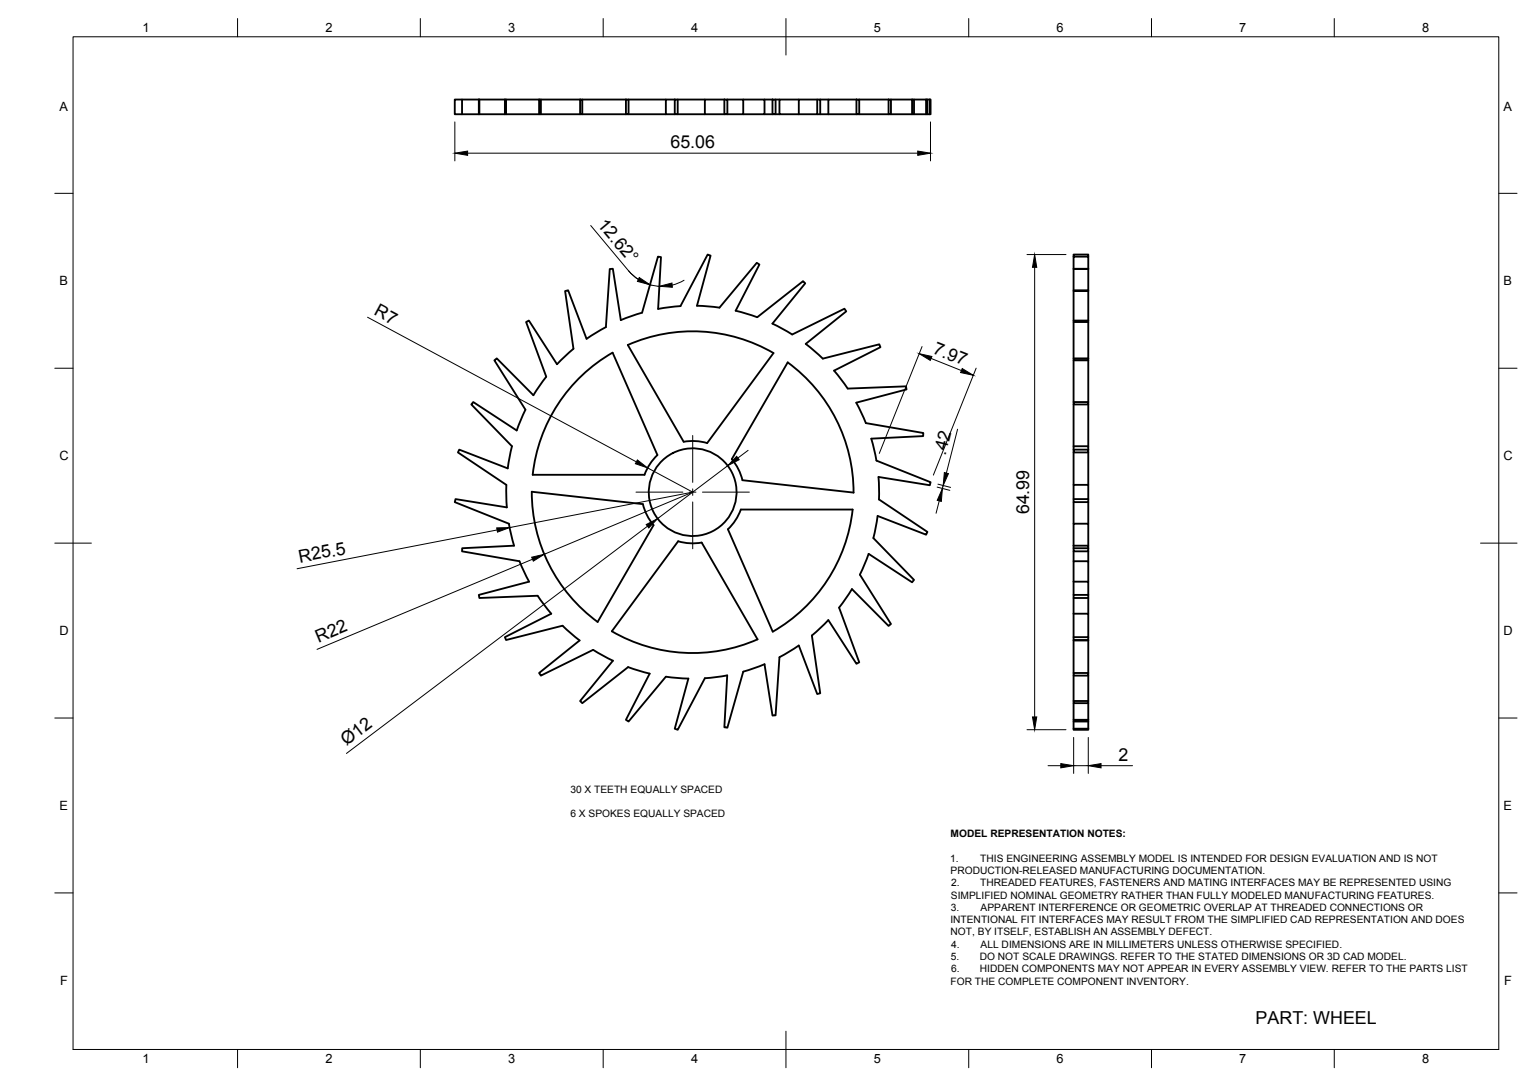
ISO-10303-21;
HEADER;
/* Generated by software containing ST-Developer
 * from STEP Tools, Inc. (www.steptools.com) 
 */

FILE_DESCRIPTION(
/* description */ (''),
/* implementation_level */ '2;1');

FILE_NAME(
/* name */ 'Wheel.step',
/* time_stamp */ '2026-10-04T15:18:51-07:00',
/* author */ (''),
/* organization */ (''),
/* preprocessor_version */ 'ST-DEVELOPER v20.2',
/* originating_system */ 'Autodesk Translation Framework v15.15.0.0',
/* authorisation */ '');

FILE_SCHEMA (('AUTOMOTIVE_DESIGN { 1 0 10303 214 3 1 1 }'));
ENDSEC;

DATA;
#10=MECHANICAL_DESIGN_GEOMETRIC_PRESENTATION_REPRESENTATION('',(#76),#9891);
#57=SHAPE_REPRESENTATION_RELATIONSHIP('SRR','None',#9928,#65);
#65=ADVANCED_BREP_SHAPE_REPRESENTATION('',(#90),#9888);
#76=STYLED_ITEM('',(#9974),#90);
#90=MANIFOLD_SOLID_BREP('Body1',#5624);
#126=FACE_BOUND('',#1015,.T.);
#127=FACE_BOUND('',#1016,.T.);
#128=FACE_BOUND('',#1017,.T.);
#129=FACE_BOUND('',#1018,.T.);
#130=FACE_BOUND('',#1019,.T.);
#131=FACE_BOUND('',#1020,.T.);
#132=FACE_BOUND('',#1021,.T.);
#133=FACE_BOUND('',#1023,.T.);
#134=FACE_BOUND('',#1024,.T.);
#135=FACE_BOUND('',#1025,.T.);
#136=FACE_BOUND('',#1026,.T.);
#137=FACE_BOUND('',#1027,.T.);
#138=FACE_BOUND('',#1028,.T.);
#139=FACE_BOUND('',#1029,.T.);
#202=PLANE('',#5949);
#203=PLANE('',#5950);
#204=PLANE('',#5951);
#205=PLANE('',#5958);
#206=PLANE('',#5959);
#207=PLANE('',#5960);
#208=PLANE('',#5964);
#209=PLANE('',#5965);
#210=PLANE('',#5966);
#211=PLANE('',#5970);
#212=PLANE('',#5971);
#213=PLANE('',#5972);
#214=PLANE('',#5976);
#215=PLANE('',#5977);
#216=PLANE('',#5978);
#217=PLANE('',#5982);
#218=PLANE('',#5983);
#219=PLANE('',#5984);
#220=PLANE('',#5991);
#221=PLANE('',#5992);
#222=PLANE('',#5993);
#223=PLANE('',#5994);
#224=PLANE('',#5995);
#225=PLANE('',#5996);
#226=PLANE('',#6000);
#227=PLANE('',#6001);
#228=PLANE('',#6002);
#229=PLANE('',#6009);
#230=PLANE('',#6010);
#231=PLANE('',#6011);
#232=PLANE('',#6018);
#233=PLANE('',#6019);
#234=PLANE('',#6020);
#235=PLANE('',#6021);
#236=PLANE('',#6022);
#237=PLANE('',#6023);
#238=PLANE('',#6024);
#239=PLANE('',#6025);
#240=PLANE('',#6026);
#241=PLANE('',#6030);
#242=PLANE('',#6031);
#243=PLANE('',#6032);
#244=PLANE('',#6036);
#245=PLANE('',#6037);
#246=PLANE('',#6038);
#247=PLANE('',#6045);
#248=PLANE('',#6046);
#249=PLANE('',#6047);
#250=PLANE('',#6051);
#251=PLANE('',#6052);
#252=PLANE('',#6053);
#253=PLANE('',#6057);
#254=PLANE('',#6058);
#255=PLANE('',#6059);
#256=PLANE('',#6060);
#257=PLANE('',#6061);
#258=PLANE('',#6062);
#259=PLANE('',#6069);
#260=PLANE('',#6070);
#261=PLANE('',#6071);
#262=PLANE('',#6072);
#263=PLANE('',#6073);
#264=PLANE('',#6074);
#265=PLANE('',#6081);
#266=PLANE('',#6082);
#267=PLANE('',#6083);
#268=PLANE('',#6084);
#269=PLANE('',#6085);
#270=PLANE('',#6086);
#271=PLANE('',#6093);
#272=PLANE('',#6094);
#273=PLANE('',#6095);
#274=PLANE('',#6099);
#275=PLANE('',#6100);
#276=PLANE('',#6101);
#277=PLANE('',#6105);
#278=PLANE('',#6106);
#279=PLANE('',#6107);
#280=PLANE('',#6111);
#281=PLANE('',#6112);
#282=PLANE('',#6113);
#283=PLANE('',#6120);
#284=PLANE('',#6121);
#285=PLANE('',#6122);
#286=PLANE('',#6123);
#287=PLANE('',#6124);
#288=PLANE('',#6125);
#289=PLANE('',#6126);
#290=PLANE('',#6127);
#291=PLANE('',#6128);
#292=PLANE('',#6129);
#293=PLANE('',#6130);
#294=PLANE('',#6143);
#295=PLANE('',#6144);
#296=PLANE('',#6151);
#297=PLANE('',#6152);
#298=PLANE('',#6159);
#299=PLANE('',#6160);
#300=PLANE('',#6167);
#301=PLANE('',#6168);
#302=PLANE('',#6175);
#303=PLANE('',#6176);
#304=PLANE('',#6180);
#305=PLANE('',#6181);
#509=FACE_OUTER_BOUND('',#869,.T.);
#510=FACE_OUTER_BOUND('',#870,.T.);
#511=FACE_OUTER_BOUND('',#871,.T.);
#512=FACE_OUTER_BOUND('',#872,.T.);
#513=FACE_OUTER_BOUND('',#873,.T.);
#514=FACE_OUTER_BOUND('',#874,.T.);
#515=FACE_OUTER_BOUND('',#875,.T.);
#516=FACE_OUTER_BOUND('',#876,.T.);
#517=FACE_OUTER_BOUND('',#877,.T.);
#518=FACE_OUTER_BOUND('',#878,.T.);
#519=FACE_OUTER_BOUND('',#879,.T.);
#520=FACE_OUTER_BOUND('',#880,.T.);
#521=FACE_OUTER_BOUND('',#881,.T.);
#522=FACE_OUTER_BOUND('',#882,.T.);
#523=FACE_OUTER_BOUND('',#883,.T.);
#524=FACE_OUTER_BOUND('',#884,.T.);
#525=FACE_OUTER_BOUND('',#885,.T.);
#526=FACE_OUTER_BOUND('',#886,.T.);
#527=FACE_OUTER_BOUND('',#887,.T.);
#528=FACE_OUTER_BOUND('',#888,.T.);
#529=FACE_OUTER_BOUND('',#889,.T.);
#530=FACE_OUTER_BOUND('',#890,.T.);
#531=FACE_OUTER_BOUND('',#891,.T.);
#532=FACE_OUTER_BOUND('',#892,.T.);
#533=FACE_OUTER_BOUND('',#893,.T.);
#534=FACE_OUTER_BOUND('',#894,.T.);
#535=FACE_OUTER_BOUND('',#895,.T.);
#536=FACE_OUTER_BOUND('',#896,.T.);
#537=FACE_OUTER_BOUND('',#897,.T.);
#538=FACE_OUTER_BOUND('',#898,.T.);
#539=FACE_OUTER_BOUND('',#899,.T.);
#540=FACE_OUTER_BOUND('',#900,.T.);
#541=FACE_OUTER_BOUND('',#901,.T.);
#542=FACE_OUTER_BOUND('',#902,.T.);
#543=FACE_OUTER_BOUND('',#903,.T.);
#544=FACE_OUTER_BOUND('',#904,.T.);
#545=FACE_OUTER_BOUND('',#905,.T.);
#546=FACE_OUTER_BOUND('',#906,.T.);
#547=FACE_OUTER_BOUND('',#907,.T.);
#548=FACE_OUTER_BOUND('',#908,.T.);
#549=FACE_OUTER_BOUND('',#909,.T.);
#550=FACE_OUTER_BOUND('',#910,.T.);
#551=FACE_OUTER_BOUND('',#911,.T.);
#552=FACE_OUTER_BOUND('',#912,.T.);
#553=FACE_OUTER_BOUND('',#913,.T.);
#554=FACE_OUTER_BOUND('',#914,.T.);
#555=FACE_OUTER_BOUND('',#915,.T.);
#556=FACE_OUTER_BOUND('',#916,.T.);
#557=FACE_OUTER_BOUND('',#917,.T.);
#558=FACE_OUTER_BOUND('',#918,.T.);
#559=FACE_OUTER_BOUND('',#919,.T.);
#560=FACE_OUTER_BOUND('',#920,.T.);
#561=FACE_OUTER_BOUND('',#921,.T.);
#562=FACE_OUTER_BOUND('',#922,.T.);
#563=FACE_OUTER_BOUND('',#923,.T.);
#564=FACE_OUTER_BOUND('',#924,.T.);
#565=FACE_OUTER_BOUND('',#925,.T.);
#566=FACE_OUTER_BOUND('',#926,.T.);
#567=FACE_OUTER_BOUND('',#927,.T.);
#568=FACE_OUTER_BOUND('',#928,.T.);
#569=FACE_OUTER_BOUND('',#929,.T.);
#570=FACE_OUTER_BOUND('',#930,.T.);
#571=FACE_OUTER_BOUND('',#931,.T.);
#572=FACE_OUTER_BOUND('',#932,.T.);
#573=FACE_OUTER_BOUND('',#933,.T.);
#574=FACE_OUTER_BOUND('',#934,.T.);
#575=FACE_OUTER_BOUND('',#935,.T.);
#576=FACE_OUTER_BOUND('',#936,.T.);
#577=FACE_OUTER_BOUND('',#937,.T.);
#578=FACE_OUTER_BOUND('',#938,.T.);
#579=FACE_OUTER_BOUND('',#939,.T.);
#580=FACE_OUTER_BOUND('',#940,.T.);
#581=FACE_OUTER_BOUND('',#941,.T.);
#582=FACE_OUTER_BOUND('',#942,.T.);
#583=FACE_OUTER_BOUND('',#943,.T.);
#584=FACE_OUTER_BOUND('',#944,.T.);
#585=FACE_OUTER_BOUND('',#945,.T.);
#586=FACE_OUTER_BOUND('',#946,.T.);
#587=FACE_OUTER_BOUND('',#947,.T.);
#588=FACE_OUTER_BOUND('',#948,.T.);
#589=FACE_OUTER_BOUND('',#949,.T.);
#590=FACE_OUTER_BOUND('',#950,.T.);
#591=FACE_OUTER_BOUND('',#951,.T.);
#592=FACE_OUTER_BOUND('',#952,.T.);
#593=FACE_OUTER_BOUND('',#953,.T.);
#594=FACE_OUTER_BOUND('',#954,.T.);
#595=FACE_OUTER_BOUND('',#955,.T.);
#596=FACE_OUTER_BOUND('',#956,.T.);
#597=FACE_OUTER_BOUND('',#957,.T.);
#598=FACE_OUTER_BOUND('',#958,.T.);
#599=FACE_OUTER_BOUND('',#959,.T.);
#600=FACE_OUTER_BOUND('',#960,.T.);
#601=FACE_OUTER_BOUND('',#961,.T.);
#602=FACE_OUTER_BOUND('',#962,.T.);
#603=FACE_OUTER_BOUND('',#963,.T.);
#604=FACE_OUTER_BOUND('',#964,.T.);
#605=FACE_OUTER_BOUND('',#965,.T.);
#606=FACE_OUTER_BOUND('',#966,.T.);
#607=FACE_OUTER_BOUND('',#967,.T.);
#608=FACE_OUTER_BOUND('',#968,.T.);
#609=FACE_OUTER_BOUND('',#969,.T.);
#610=FACE_OUTER_BOUND('',#970,.T.);
#611=FACE_OUTER_BOUND('',#971,.T.);
#612=FACE_OUTER_BOUND('',#972,.T.);
#613=FACE_OUTER_BOUND('',#973,.T.);
#614=FACE_OUTER_BOUND('',#974,.T.);
#615=FACE_OUTER_BOUND('',#975,.T.);
#616=FACE_OUTER_BOUND('',#976,.T.);
#617=FACE_OUTER_BOUND('',#977,.T.);
#618=FACE_OUTER_BOUND('',#978,.T.);
#619=FACE_OUTER_BOUND('',#979,.T.);
#620=FACE_OUTER_BOUND('',#980,.T.);
#621=FACE_OUTER_BOUND('',#981,.T.);
#622=FACE_OUTER_BOUND('',#982,.T.);
#623=FACE_OUTER_BOUND('',#983,.T.);
#624=FACE_OUTER_BOUND('',#984,.T.);
#625=FACE_OUTER_BOUND('',#985,.T.);
#626=FACE_OUTER_BOUND('',#986,.T.);
#627=FACE_OUTER_BOUND('',#987,.T.);
#628=FACE_OUTER_BOUND('',#988,.T.);
#629=FACE_OUTER_BOUND('',#989,.T.);
#630=FACE_OUTER_BOUND('',#990,.T.);
#631=FACE_OUTER_BOUND('',#991,.T.);
#632=FACE_OUTER_BOUND('',#992,.T.);
#633=FACE_OUTER_BOUND('',#993,.T.);
#634=FACE_OUTER_BOUND('',#994,.T.);
#635=FACE_OUTER_BOUND('',#995,.T.);
#636=FACE_OUTER_BOUND('',#996,.T.);
#637=FACE_OUTER_BOUND('',#997,.T.);
#638=FACE_OUTER_BOUND('',#998,.T.);
#639=FACE_OUTER_BOUND('',#999,.T.);
#640=FACE_OUTER_BOUND('',#1000,.T.);
#641=FACE_OUTER_BOUND('',#1001,.T.);
#642=FACE_OUTER_BOUND('',#1002,.T.);
#643=FACE_OUTER_BOUND('',#1003,.T.);
#644=FACE_OUTER_BOUND('',#1004,.T.);
#645=FACE_OUTER_BOUND('',#1005,.T.);
#646=FACE_OUTER_BOUND('',#1006,.T.);
#647=FACE_OUTER_BOUND('',#1007,.T.);
#648=FACE_OUTER_BOUND('',#1008,.T.);
#649=FACE_OUTER_BOUND('',#1009,.T.);
#650=FACE_OUTER_BOUND('',#1010,.T.);
#651=FACE_OUTER_BOUND('',#1011,.T.);
#652=FACE_OUTER_BOUND('',#1012,.T.);
#653=FACE_OUTER_BOUND('',#1013,.T.);
#654=FACE_OUTER_BOUND('',#1014,.T.);
#655=FACE_OUTER_BOUND('',#1022,.T.);
#869=EDGE_LOOP('',(#4016,#4017,#4018,#4019));
#870=EDGE_LOOP('',(#4020,#4021,#4022,#4023));
#871=EDGE_LOOP('',(#4024,#4025,#4026,#4027));
#872=EDGE_LOOP('',(#4028,#4029,#4030,#4031));
#873=EDGE_LOOP('',(#4032,#4033,#4034,#4035));
#874=EDGE_LOOP('',(#4036,#4037,#4038,#4039));
#875=EDGE_LOOP('',(#4040,#4041,#4042,#4043));
#876=EDGE_LOOP('',(#4044,#4045,#4046,#4047));
#877=EDGE_LOOP('',(#4048,#4049,#4050,#4051));
#878=EDGE_LOOP('',(#4052,#4053,#4054,#4055));
#879=EDGE_LOOP('',(#4056,#4057,#4058,#4059));
#880=EDGE_LOOP('',(#4060,#4061,#4062,#4063));
#881=EDGE_LOOP('',(#4064,#4065,#4066,#4067));
#882=EDGE_LOOP('',(#4068,#4069,#4070,#4071));
#883=EDGE_LOOP('',(#4072,#4073,#4074,#4075));
#884=EDGE_LOOP('',(#4076,#4077,#4078,#4079));
#885=EDGE_LOOP('',(#4080,#4081,#4082,#4083));
#886=EDGE_LOOP('',(#4084,#4085,#4086,#4087));
#887=EDGE_LOOP('',(#4088,#4089,#4090,#4091));
#888=EDGE_LOOP('',(#4092,#4093,#4094,#4095));
#889=EDGE_LOOP('',(#4096,#4097,#4098,#4099));
#890=EDGE_LOOP('',(#4100,#4101,#4102,#4103));
#891=EDGE_LOOP('',(#4104,#4105,#4106,#4107));
#892=EDGE_LOOP('',(#4108,#4109,#4110,#4111));
#893=EDGE_LOOP('',(#4112,#4113,#4114,#4115));
#894=EDGE_LOOP('',(#4116,#4117,#4118,#4119));
#895=EDGE_LOOP('',(#4120,#4121,#4122,#4123));
#896=EDGE_LOOP('',(#4124,#4125,#4126,#4127));
#897=EDGE_LOOP('',(#4128,#4129,#4130,#4131));
#898=EDGE_LOOP('',(#4132,#4133,#4134,#4135));
#899=EDGE_LOOP('',(#4136,#4137,#4138,#4139));
#900=EDGE_LOOP('',(#4140,#4141,#4142,#4143));
#901=EDGE_LOOP('',(#4144,#4145,#4146,#4147));
#902=EDGE_LOOP('',(#4148,#4149,#4150,#4151));
#903=EDGE_LOOP('',(#4152,#4153,#4154,#4155));
#904=EDGE_LOOP('',(#4156,#4157,#4158,#4159));
#905=EDGE_LOOP('',(#4160,#4161,#4162,#4163));
#906=EDGE_LOOP('',(#4164,#4165,#4166,#4167));
#907=EDGE_LOOP('',(#4168,#4169,#4170,#4171));
#908=EDGE_LOOP('',(#4172,#4173,#4174,#4175));
#909=EDGE_LOOP('',(#4176,#4177,#4178,#4179));
#910=EDGE_LOOP('',(#4180,#4181,#4182,#4183));
#911=EDGE_LOOP('',(#4184,#4185,#4186,#4187));
#912=EDGE_LOOP('',(#4188,#4189,#4190,#4191));
#913=EDGE_LOOP('',(#4192,#4193,#4194,#4195));
#914=EDGE_LOOP('',(#4196,#4197,#4198,#4199));
#915=EDGE_LOOP('',(#4200,#4201,#4202,#4203));
#916=EDGE_LOOP('',(#4204,#4205,#4206,#4207));
#917=EDGE_LOOP('',(#4208,#4209,#4210,#4211));
#918=EDGE_LOOP('',(#4212,#4213,#4214,#4215));
#919=EDGE_LOOP('',(#4216,#4217,#4218,#4219));
#920=EDGE_LOOP('',(#4220,#4221,#4222,#4223));
#921=EDGE_LOOP('',(#4224,#4225,#4226,#4227));
#922=EDGE_LOOP('',(#4228,#4229,#4230,#4231));
#923=EDGE_LOOP('',(#4232,#4233,#4234,#4235));
#924=EDGE_LOOP('',(#4236,#4237,#4238,#4239));
#925=EDGE_LOOP('',(#4240,#4241,#4242,#4243));
#926=EDGE_LOOP('',(#4244,#4245,#4246,#4247));
#927=EDGE_LOOP('',(#4248,#4249,#4250,#4251));
#928=EDGE_LOOP('',(#4252,#4253,#4254,#4255));
#929=EDGE_LOOP('',(#4256,#4257,#4258,#4259));
#930=EDGE_LOOP('',(#4260,#4261,#4262,#4263));
#931=EDGE_LOOP('',(#4264,#4265,#4266,#4267));
#932=EDGE_LOOP('',(#4268,#4269,#4270,#4271));
#933=EDGE_LOOP('',(#4272,#4273,#4274,#4275));
#934=EDGE_LOOP('',(#4276,#4277,#4278,#4279));
#935=EDGE_LOOP('',(#4280,#4281,#4282,#4283));
#936=EDGE_LOOP('',(#4284,#4285,#4286,#4287));
#937=EDGE_LOOP('',(#4288,#4289,#4290,#4291));
#938=EDGE_LOOP('',(#4292,#4293,#4294,#4295));
#939=EDGE_LOOP('',(#4296,#4297,#4298,#4299));
#940=EDGE_LOOP('',(#4300,#4301,#4302,#4303));
#941=EDGE_LOOP('',(#4304,#4305,#4306,#4307));
#942=EDGE_LOOP('',(#4308,#4309,#4310,#4311));
#943=EDGE_LOOP('',(#4312,#4313,#4314,#4315));
#944=EDGE_LOOP('',(#4316,#4317,#4318,#4319));
#945=EDGE_LOOP('',(#4320,#4321,#4322,#4323));
#946=EDGE_LOOP('',(#4324,#4325,#4326,#4327));
#947=EDGE_LOOP('',(#4328,#4329,#4330,#4331));
#948=EDGE_LOOP('',(#4332,#4333,#4334,#4335));
#949=EDGE_LOOP('',(#4336,#4337,#4338,#4339));
#950=EDGE_LOOP('',(#4340,#4341,#4342,#4343));
#951=EDGE_LOOP('',(#4344,#4345,#4346,#4347));
#952=EDGE_LOOP('',(#4348,#4349,#4350,#4351));
#953=EDGE_LOOP('',(#4352,#4353,#4354,#4355));
#954=EDGE_LOOP('',(#4356,#4357,#4358,#4359));
#955=EDGE_LOOP('',(#4360,#4361,#4362,#4363));
#956=EDGE_LOOP('',(#4364,#4365,#4366,#4367));
#957=EDGE_LOOP('',(#4368,#4369,#4370,#4371));
#958=EDGE_LOOP('',(#4372,#4373,#4374,#4375));
#959=EDGE_LOOP('',(#4376,#4377,#4378,#4379));
#960=EDGE_LOOP('',(#4380,#4381,#4382,#4383));
#961=EDGE_LOOP('',(#4384,#4385,#4386,#4387));
#962=EDGE_LOOP('',(#4388,#4389,#4390,#4391));
#963=EDGE_LOOP('',(#4392,#4393,#4394,#4395));
#964=EDGE_LOOP('',(#4396,#4397,#4398,#4399));
#965=EDGE_LOOP('',(#4400,#4401,#4402,#4403));
#966=EDGE_LOOP('',(#4404,#4405,#4406,#4407));
#967=EDGE_LOOP('',(#4408,#4409,#4410,#4411));
#968=EDGE_LOOP('',(#4412,#4413,#4414,#4415));
#969=EDGE_LOOP('',(#4416,#4417,#4418,#4419));
#970=EDGE_LOOP('',(#4420,#4421,#4422,#4423));
#971=EDGE_LOOP('',(#4424,#4425,#4426,#4427));
#972=EDGE_LOOP('',(#4428,#4429,#4430,#4431));
#973=EDGE_LOOP('',(#4432,#4433,#4434,#4435));
#974=EDGE_LOOP('',(#4436,#4437,#4438,#4439));
#975=EDGE_LOOP('',(#4440,#4441,#4442,#4443));
#976=EDGE_LOOP('',(#4444,#4445,#4446,#4447));
#977=EDGE_LOOP('',(#4448,#4449,#4450,#4451));
#978=EDGE_LOOP('',(#4452,#4453,#4454,#4455));
#979=EDGE_LOOP('',(#4456,#4457,#4458,#4459));
#980=EDGE_LOOP('',(#4460,#4461,#4462,#4463));
#981=EDGE_LOOP('',(#4464,#4465,#4466,#4467));
#982=EDGE_LOOP('',(#4468,#4469,#4470,#4471));
#983=EDGE_LOOP('',(#4472,#4473,#4474,#4475));
#984=EDGE_LOOP('',(#4476,#4477,#4478,#4479));
#985=EDGE_LOOP('',(#4480,#4481,#4482,#4483));
#986=EDGE_LOOP('',(#4484,#4485,#4486,#4487));
#987=EDGE_LOOP('',(#4488,#4489,#4490,#4491));
#988=EDGE_LOOP('',(#4492,#4493,#4494,#4495));
#989=EDGE_LOOP('',(#4496,#4497,#4498,#4499));
#990=EDGE_LOOP('',(#4500,#4501,#4502,#4503));
#991=EDGE_LOOP('',(#4504,#4505,#4506,#4507));
#992=EDGE_LOOP('',(#4508,#4509,#4510,#4511));
#993=EDGE_LOOP('',(#4512,#4513,#4514,#4515));
#994=EDGE_LOOP('',(#4516,#4517,#4518,#4519));
#995=EDGE_LOOP('',(#4520,#4521,#4522,#4523));
#996=EDGE_LOOP('',(#4524,#4525,#4526,#4527));
#997=EDGE_LOOP('',(#4528,#4529,#4530,#4531));
#998=EDGE_LOOP('',(#4532,#4533,#4534,#4535));
#999=EDGE_LOOP('',(#4536,#4537,#4538,#4539));
#1000=EDGE_LOOP('',(#4540,#4541,#4542,#4543));
#1001=EDGE_LOOP('',(#4544,#4545,#4546,#4547));
#1002=EDGE_LOOP('',(#4548,#4549,#4550,#4551));
#1003=EDGE_LOOP('',(#4552,#4553,#4554,#4555));
#1004=EDGE_LOOP('',(#4556,#4557,#4558,#4559));
#1005=EDGE_LOOP('',(#4560,#4561,#4562,#4563));
#1006=EDGE_LOOP('',(#4564,#4565,#4566,#4567));
#1007=EDGE_LOOP('',(#4568,#4569,#4570,#4571));
#1008=EDGE_LOOP('',(#4572,#4573,#4574,#4575));
#1009=EDGE_LOOP('',(#4576,#4577,#4578,#4579));
#1010=EDGE_LOOP('',(#4580,#4581,#4582,#4583));
#1011=EDGE_LOOP('',(#4584,#4585,#4586,#4587));
#1012=EDGE_LOOP('',(#4588,#4589,#4590,#4591));
#1013=EDGE_LOOP('',(#4592,#4593,#4594,#4595));
#1014=EDGE_LOOP('',(#4596,#4597,#4598,#4599,#4600,#4601,#4602,#4603,#4604,
#4605,#4606,#4607,#4608,#4609,#4610,#4611,#4612,#4613,#4614,#4615,#4616,
#4617,#4618,#4619,#4620,#4621,#4622,#4623,#4624,#4625,#4626,#4627,#4628,
#4629,#4630,#4631,#4632,#4633,#4634,#4635,#4636,#4637,#4638,#4639,#4640,
#4641,#4642,#4643,#4644,#4645,#4646,#4647,#4648,#4649,#4650,#4651,#4652,
#4653,#4654,#4655,#4656,#4657,#4658,#4659,#4660,#4661,#4662,#4663,#4664,
#4665,#4666,#4667,#4668,#4669,#4670,#4671,#4672,#4673,#4674,#4675,#4676,
#4677,#4678,#4679,#4680,#4681,#4682,#4683,#4684,#4685,#4686,#4687,#4688,
#4689,#4690,#4691,#4692,#4693,#4694,#4695,#4696,#4697,#4698,#4699,#4700,
#4701,#4702,#4703,#4704,#4705,#4706,#4707,#4708,#4709,#4710,#4711,#4712,
#4713,#4714,#4715));
#1015=EDGE_LOOP('',(#4716,#4717,#4718,#4719));
#1016=EDGE_LOOP('',(#4720,#4721,#4722,#4723));
#1017=EDGE_LOOP('',(#4724,#4725,#4726,#4727));
#1018=EDGE_LOOP('',(#4728,#4729,#4730,#4731));
#1019=EDGE_LOOP('',(#4732,#4733,#4734,#4735));
#1020=EDGE_LOOP('',(#4736));
#1021=EDGE_LOOP('',(#4737,#4738,#4739,#4740));
#1022=EDGE_LOOP('',(#4741,#4742,#4743,#4744,#4745,#4746,#4747,#4748,#4749,
#4750,#4751,#4752,#4753,#4754,#4755,#4756,#4757,#4758,#4759,#4760,#4761,
#4762,#4763,#4764,#4765,#4766,#4767,#4768,#4769,#4770,#4771,#4772,#4773,
#4774,#4775,#4776,#4777,#4778,#4779,#4780,#4781,#4782,#4783,#4784,#4785,
#4786,#4787,#4788,#4789,#4790,#4791,#4792,#4793,#4794,#4795,#4796,#4797,
#4798,#4799,#4800,#4801,#4802,#4803,#4804,#4805,#4806,#4807,#4808,#4809,
#4810,#4811,#4812,#4813,#4814,#4815,#4816,#4817,#4818,#4819,#4820,#4821,
#4822,#4823,#4824,#4825,#4826,#4827,#4828,#4829,#4830,#4831,#4832,#4833,
#4834,#4835,#4836,#4837,#4838,#4839,#4840,#4841,#4842,#4843,#4844,#4845,
#4846,#4847,#4848,#4849,#4850,#4851,#4852,#4853,#4854,#4855,#4856,#4857,
#4858,#4859,#4860));
#1023=EDGE_LOOP('',(#4861,#4862,#4863,#4864));
#1024=EDGE_LOOP('',(#4865,#4866,#4867,#4868));
#1025=EDGE_LOOP('',(#4869,#4870,#4871,#4872));
#1026=EDGE_LOOP('',(#4873,#4874,#4875,#4876));
#1027=EDGE_LOOP('',(#4877,#4878,#4879,#4880));
#1028=EDGE_LOOP('',(#4881));
#1029=EDGE_LOOP('',(#4882,#4883,#4884,#4885));
#1187=LINE('',#8656,#1651);
#1188=LINE('',#8658,#1652);
#1189=LINE('',#8660,#1653);
#1190=LINE('',#8661,#1654);
#1191=LINE('',#8664,#1655);
#1192=LINE('',#8666,#1656);
#1193=LINE('',#8667,#1657);
#1194=LINE('',#8670,#1658);
#1195=LINE('',#8672,#1659);
#1196=LINE('',#8673,#1660);
#1197=LINE('',#8678,#1661);
#1198=LINE('',#8684,#1662);
#1199=LINE('',#8689,#1663);
#1200=LINE('',#8691,#1664);
#1201=LINE('',#8693,#1665);
#1202=LINE('',#8694,#1666);
#1203=LINE('',#8697,#1667);
#1204=LINE('',#8699,#1668);
#1205=LINE('',#8700,#1669);
#1206=LINE('',#8702,#1670);
#1207=LINE('',#8703,#1671);
#1208=LINE('',#8708,#1672);
#1209=LINE('',#8713,#1673);
#1210=LINE('',#8715,#1674);
#1211=LINE('',#8717,#1675);
#1212=LINE('',#8718,#1676);
#1213=LINE('',#8721,#1677);
#1214=LINE('',#8723,#1678);
#1215=LINE('',#8724,#1679);
#1216=LINE('',#8726,#1680);
#1217=LINE('',#8727,#1681);
#1218=LINE('',#8732,#1682);
#1219=LINE('',#8737,#1683);
#1220=LINE('',#8739,#1684);
#1221=LINE('',#8741,#1685);
#1222=LINE('',#8742,#1686);
#1223=LINE('',#8745,#1687);
#1224=LINE('',#8747,#1688);
#1225=LINE('',#8748,#1689);
#1226=LINE('',#8750,#1690);
#1227=LINE('',#8751,#1691);
#1228=LINE('',#8756,#1692);
#1229=LINE('',#8761,#1693);
#1230=LINE('',#8763,#1694);
#1231=LINE('',#8765,#1695);
#1232=LINE('',#8766,#1696);
#1233=LINE('',#8769,#1697);
#1234=LINE('',#8771,#1698);
#1235=LINE('',#8772,#1699);
#1236=LINE('',#8774,#1700);
#1237=LINE('',#8775,#1701);
#1238=LINE('',#8780,#1702);
#1239=LINE('',#8785,#1703);
#1240=LINE('',#8787,#1704);
#1241=LINE('',#8789,#1705);
#1242=LINE('',#8790,#1706);
#1243=LINE('',#8793,#1707);
#1244=LINE('',#8795,#1708);
#1245=LINE('',#8796,#1709);
#1246=LINE('',#8799,#1710);
#1247=LINE('',#8801,#1711);
#1248=LINE('',#8802,#1712);
#1249=LINE('',#8807,#1713);
#1250=LINE('',#8813,#1714);
#1251=LINE('',#8818,#1715);
#1252=LINE('',#8820,#1716);
#1253=LINE('',#8822,#1717);
#1254=LINE('',#8823,#1718);
#1255=LINE('',#8825,#1719);
#1256=LINE('',#8826,#1720);
#1257=LINE('',#8828,#1721);
#1258=LINE('',#8829,#1722);
#1259=LINE('',#8833,#1723);
#1260=LINE('',#8835,#1724);
#1261=LINE('',#8837,#1725);
#1262=LINE('',#8838,#1726);
#1263=LINE('',#8841,#1727);
#1264=LINE('',#8843,#1728);
#1265=LINE('',#8844,#1729);
#1266=LINE('',#8846,#1730);
#1267=LINE('',#8847,#1731);
#1268=LINE('',#8852,#1732);
#1269=LINE('',#8857,#1733);
#1270=LINE('',#8859,#1734);
#1271=LINE('',#8861,#1735);
#1272=LINE('',#8862,#1736);
#1273=LINE('',#8865,#1737);
#1274=LINE('',#8867,#1738);
#1275=LINE('',#8868,#1739);
#1276=LINE('',#8871,#1740);
#1277=LINE('',#8873,#1741);
#1278=LINE('',#8874,#1742);
#1279=LINE('',#8879,#1743);
#1280=LINE('',#8885,#1744);
#1281=LINE('',#8890,#1745);
#1282=LINE('',#8892,#1746);
#1283=LINE('',#8894,#1747);
#1284=LINE('',#8895,#1748);
#1285=LINE('',#8898,#1749);
#1286=LINE('',#8900,#1750);
#1287=LINE('',#8901,#1751);
#1288=LINE('',#8904,#1752);
#1289=LINE('',#8906,#1753);
#1290=LINE('',#8907,#1754);
#1291=LINE('',#8912,#1755);
#1292=LINE('',#8918,#1756);
#1293=LINE('',#8923,#1757);
#1294=LINE('',#8925,#1758);
#1295=LINE('',#8927,#1759);
#1296=LINE('',#8928,#1760);
#1297=LINE('',#8930,#1761);
#1298=LINE('',#8931,#1762);
#1299=LINE('',#8933,#1763);
#1300=LINE('',#8934,#1764);
#1301=LINE('',#8938,#1765);
#1302=LINE('',#8940,#1766);
#1303=LINE('',#8942,#1767);
#1304=LINE('',#8943,#1768);
#1305=LINE('',#8945,#1769);
#1306=LINE('',#8946,#1770);
#1307=LINE('',#8948,#1771);
#1308=LINE('',#8949,#1772);
#1309=LINE('',#8953,#1773);
#1310=LINE('',#8955,#1774);
#1311=LINE('',#8957,#1775);
#1312=LINE('',#8958,#1776);
#1313=LINE('',#8961,#1777);
#1314=LINE('',#8963,#1778);
#1315=LINE('',#8964,#1779);
#1316=LINE('',#8966,#1780);
#1317=LINE('',#8967,#1781);
#1318=LINE('',#8972,#1782);
#1319=LINE('',#8977,#1783);
#1320=LINE('',#8979,#1784);
#1321=LINE('',#8981,#1785);
#1322=LINE('',#8982,#1786);
#1323=LINE('',#8985,#1787);
#1324=LINE('',#8987,#1788);
#1325=LINE('',#8988,#1789);
#1326=LINE('',#8990,#1790);
#1327=LINE('',#8991,#1791);
#1328=LINE('',#8996,#1792);
#1329=LINE('',#9001,#1793);
#1330=LINE('',#9003,#1794);
#1331=LINE('',#9005,#1795);
#1332=LINE('',#9006,#1796);
#1333=LINE('',#9009,#1797);
#1334=LINE('',#9011,#1798);
#1335=LINE('',#9012,#1799);
#1336=LINE('',#9015,#1800);
#1337=LINE('',#9017,#1801);
#1338=LINE('',#9018,#1802);
#1339=LINE('',#9023,#1803);
#1340=LINE('',#9029,#1804);
#1341=LINE('',#9034,#1805);
#1342=LINE('',#9036,#1806);
#1343=LINE('',#9038,#1807);
#1344=LINE('',#9039,#1808);
#1345=LINE('',#9042,#1809);
#1346=LINE('',#9044,#1810);
#1347=LINE('',#9045,#1811);
#1348=LINE('',#9047,#1812);
#1349=LINE('',#9048,#1813);
#1350=LINE('',#9053,#1814);
#1351=LINE('',#9058,#1815);
#1352=LINE('',#9060,#1816);
#1353=LINE('',#9062,#1817);
#1354=LINE('',#9063,#1818);
#1355=LINE('',#9066,#1819);
#1356=LINE('',#9068,#1820);
#1357=LINE('',#9069,#1821);
#1358=LINE('',#9071,#1822);
#1359=LINE('',#9072,#1823);
#1360=LINE('',#9077,#1824);
#1361=LINE('',#9082,#1825);
#1362=LINE('',#9084,#1826);
#1363=LINE('',#9086,#1827);
#1364=LINE('',#9087,#1828);
#1365=LINE('',#9089,#1829);
#1366=LINE('',#9090,#1830);
#1367=LINE('',#9092,#1831);
#1368=LINE('',#9093,#1832);
#1369=LINE('',#9097,#1833);
#1370=LINE('',#9099,#1834);
#1371=LINE('',#9101,#1835);
#1372=LINE('',#9102,#1836);
#1373=LINE('',#9105,#1837);
#1374=LINE('',#9107,#1838);
#1375=LINE('',#9108,#1839);
#1376=LINE('',#9111,#1840);
#1377=LINE('',#9113,#1841);
#1378=LINE('',#9114,#1842);
#1379=LINE('',#9119,#1843);
#1380=LINE('',#9125,#1844);
#1381=LINE('',#9130,#1845);
#1382=LINE('',#9132,#1846);
#1383=LINE('',#9134,#1847);
#1384=LINE('',#9135,#1848);
#1385=LINE('',#9137,#1849);
#1386=LINE('',#9138,#1850);
#1387=LINE('',#9140,#1851);
#1388=LINE('',#9141,#1852);
#1389=LINE('',#9145,#1853);
#1390=LINE('',#9147,#1854);
#1391=LINE('',#9149,#1855);
#1392=LINE('',#9150,#1856);
#1393=LINE('',#9153,#1857);
#1394=LINE('',#9155,#1858);
#1395=LINE('',#9156,#1859);
#1396=LINE('',#9159,#1860);
#1397=LINE('',#9161,#1861);
#1398=LINE('',#9162,#1862);
#1399=LINE('',#9167,#1863);
#1400=LINE('',#9173,#1864);
#1401=LINE('',#9178,#1865);
#1402=LINE('',#9180,#1866);
#1403=LINE('',#9182,#1867);
#1404=LINE('',#9183,#1868);
#1405=LINE('',#9185,#1869);
#1406=LINE('',#9186,#1870);
#1407=LINE('',#9188,#1871);
#1408=LINE('',#9189,#1872);
#1409=LINE('',#9193,#1873);
#1410=LINE('',#9195,#1874);
#1411=LINE('',#9197,#1875);
#1412=LINE('',#9198,#1876);
#1413=LINE('',#9201,#1877);
#1414=LINE('',#9203,#1878);
#1415=LINE('',#9204,#1879);
#1416=LINE('',#9207,#1880);
#1417=LINE('',#9209,#1881);
#1418=LINE('',#9210,#1882);
#1419=LINE('',#9215,#1883);
#1420=LINE('',#9221,#1884);
#1421=LINE('',#9226,#1885);
#1422=LINE('',#9228,#1886);
#1423=LINE('',#9230,#1887);
#1424=LINE('',#9231,#1888);
#1425=LINE('',#9234,#1889);
#1426=LINE('',#9236,#1890);
#1427=LINE('',#9237,#1891);
#1428=LINE('',#9239,#1892);
#1429=LINE('',#9240,#1893);
#1430=LINE('',#9245,#1894);
#1431=LINE('',#9250,#1895);
#1432=LINE('',#9252,#1896);
#1433=LINE('',#9254,#1897);
#1434=LINE('',#9255,#1898);
#1435=LINE('',#9258,#1899);
#1436=LINE('',#9260,#1900);
#1437=LINE('',#9261,#1901);
#1438=LINE('',#9263,#1902);
#1439=LINE('',#9264,#1903);
#1440=LINE('',#9269,#1904);
#1441=LINE('',#9274,#1905);
#1442=LINE('',#9276,#1906);
#1443=LINE('',#9278,#1907);
#1444=LINE('',#9279,#1908);
#1445=LINE('',#9281,#1909);
#1446=LINE('',#9282,#1910);
#1447=LINE('',#9285,#1911);
#1448=LINE('',#9287,#1912);
#1449=LINE('',#9288,#1913);
#1450=LINE('',#9293,#1914);
#1451=LINE('',#9298,#1915);
#1452=LINE('',#9300,#1916);
#1453=LINE('',#9302,#1917);
#1454=LINE('',#9303,#1918);
#1455=LINE('',#9306,#1919);
#1456=LINE('',#9308,#1920);
#1457=LINE('',#9309,#1921);
#1458=LINE('',#9312,#1922);
#1459=LINE('',#9314,#1923);
#1460=LINE('',#9315,#1924);
#1461=LINE('',#9320,#1925);
#1462=LINE('',#9326,#1926);
#1463=LINE('',#9331,#1927);
#1464=LINE('',#9333,#1928);
#1465=LINE('',#9335,#1929);
#1466=LINE('',#9336,#1930);
#1467=LINE('',#9338,#1931);
#1468=LINE('',#9339,#1932);
#1469=LINE('',#9341,#1933);
#1470=LINE('',#9342,#1934);
#1471=LINE('',#9346,#1935);
#1472=LINE('',#9348,#1936);
#1473=LINE('',#9350,#1937);
#1474=LINE('',#9351,#1938);
#1475=LINE('',#9353,#1939);
#1476=LINE('',#9354,#1940);
#1477=LINE('',#9356,#1941);
#1478=LINE('',#9357,#1942);
#1479=LINE('',#9361,#1943);
#1480=LINE('',#9363,#1944);
#1481=LINE('',#9365,#1945);
#1482=LINE('',#9366,#1946);
#1483=LINE('',#9368,#1947);
#1484=LINE('',#9369,#1948);
#1485=LINE('',#9371,#1949);
#1486=LINE('',#9372,#1950);
#1487=LINE('',#9376,#1951);
#1488=LINE('',#9378,#1952);
#1489=LINE('',#9380,#1953);
#1490=LINE('',#9381,#1954);
#1491=LINE('',#9385,#1955);
#1492=LINE('',#9387,#1956);
#1493=LINE('',#9389,#1957);
#1494=LINE('',#9390,#1958);
#1495=LINE('',#9395,#1959);
#1496=LINE('',#9401,#1960);
#1497=LINE('',#9407,#1961);
#1498=LINE('',#9413,#1962);
#1499=LINE('',#9416,#1963);
#1500=LINE('',#9417,#1964);
#1501=LINE('',#9421,#1965);
#1502=LINE('',#9423,#1966);
#1503=LINE('',#9425,#1967);
#1504=LINE('',#9426,#1968);
#1505=LINE('',#9431,#1969);
#1506=LINE('',#9437,#1970);
#1507=LINE('',#9440,#1971);
#1508=LINE('',#9441,#1972);
#1509=LINE('',#9445,#1973);
#1510=LINE('',#9447,#1974);
#1511=LINE('',#9449,#1975);
#1512=LINE('',#9450,#1976);
#1513=LINE('',#9455,#1977);
#1514=LINE('',#9461,#1978);
#1515=LINE('',#9464,#1979);
#1516=LINE('',#9465,#1980);
#1517=LINE('',#9469,#1981);
#1518=LINE('',#9471,#1982);
#1519=LINE('',#9473,#1983);
#1520=LINE('',#9474,#1984);
#1521=LINE('',#9479,#1985);
#1522=LINE('',#9485,#1986);
#1523=LINE('',#9488,#1987);
#1524=LINE('',#9489,#1988);
#1525=LINE('',#9493,#1989);
#1526=LINE('',#9495,#1990);
#1527=LINE('',#9497,#1991);
#1528=LINE('',#9498,#1992);
#1529=LINE('',#9503,#1993);
#1530=LINE('',#9509,#1994);
#1531=LINE('',#9512,#1995);
#1532=LINE('',#9513,#1996);
#1533=LINE('',#9515,#1997);
#1534=LINE('',#9516,#1998);
#1535=LINE('',#9521,#1999);
#1651=VECTOR('',#6888,10.);
#1652=VECTOR('',#6889,10.);
#1653=VECTOR('',#6890,10.);
#1654=VECTOR('',#6891,10.);
#1655=VECTOR('',#6894,10.);
#1656=VECTOR('',#6895,10.);
#1657=VECTOR('',#6896,10.);
#1658=VECTOR('',#6899,10.);
#1659=VECTOR('',#6900,10.);
#1660=VECTOR('',#6901,10.);
#1661=VECTOR('',#6906,10.);
#1662=VECTOR('',#6913,10.);
#1663=VECTOR('',#6918,10.);
#1664=VECTOR('',#6919,10.);
#1665=VECTOR('',#6920,10.);
#1666=VECTOR('',#6921,10.);
#1667=VECTOR('',#6924,10.);
#1668=VECTOR('',#6925,10.);
#1669=VECTOR('',#6926,10.);
#1670=VECTOR('',#6929,10.);
#1671=VECTOR('',#6930,10.);
#1672=VECTOR('',#6935,10.);
#1673=VECTOR('',#6940,10.);
#1674=VECTOR('',#6941,10.);
#1675=VECTOR('',#6942,10.);
#1676=VECTOR('',#6943,10.);
#1677=VECTOR('',#6946,10.);
#1678=VECTOR('',#6947,10.);
#1679=VECTOR('',#6948,10.);
#1680=VECTOR('',#6951,10.);
#1681=VECTOR('',#6952,10.);
#1682=VECTOR('',#6957,10.);
#1683=VECTOR('',#6962,10.);
#1684=VECTOR('',#6963,10.);
#1685=VECTOR('',#6964,10.);
#1686=VECTOR('',#6965,10.);
#1687=VECTOR('',#6968,10.);
#1688=VECTOR('',#6969,10.);
#1689=VECTOR('',#6970,10.);
#1690=VECTOR('',#6973,10.);
#1691=VECTOR('',#6974,10.);
#1692=VECTOR('',#6979,10.);
#1693=VECTOR('',#6984,10.);
#1694=VECTOR('',#6985,10.);
#1695=VECTOR('',#6986,10.);
#1696=VECTOR('',#6987,10.);
#1697=VECTOR('',#6990,10.);
#1698=VECTOR('',#6991,10.);
#1699=VECTOR('',#6992,10.);
#1700=VECTOR('',#6995,9.99999999999999);
#1701=VECTOR('',#6996,9.99999999999999);
#1702=VECTOR('',#7001,10.);
#1703=VECTOR('',#7006,10.);
#1704=VECTOR('',#7007,10.);
#1705=VECTOR('',#7008,10.);
#1706=VECTOR('',#7009,10.);
#1707=VECTOR('',#7012,10.);
#1708=VECTOR('',#7013,10.);
#1709=VECTOR('',#7014,10.);
#1710=VECTOR('',#7017,10.);
#1711=VECTOR('',#7018,10.);
#1712=VECTOR('',#7019,10.);
#1713=VECTOR('',#7024,10.);
#1714=VECTOR('',#7031,10.);
#1715=VECTOR('',#7036,9.99999999999999);
#1716=VECTOR('',#7037,10.);
#1717=VECTOR('',#7038,9.99999999999999);
#1718=VECTOR('',#7039,10.);
#1719=VECTOR('',#7042,10.);
#1720=VECTOR('',#7043,10.);
#1721=VECTOR('',#7046,10.);
#1722=VECTOR('',#7047,10.);
#1723=VECTOR('',#7050,10.);
#1724=VECTOR('',#7051,10.);
#1725=VECTOR('',#7052,10.);
#1726=VECTOR('',#7053,10.);
#1727=VECTOR('',#7056,10.);
#1728=VECTOR('',#7057,10.);
#1729=VECTOR('',#7058,10.);
#1730=VECTOR('',#7061,10.);
#1731=VECTOR('',#7062,10.);
#1732=VECTOR('',#7067,10.);
#1733=VECTOR('',#7072,10.);
#1734=VECTOR('',#7073,10.);
#1735=VECTOR('',#7074,10.);
#1736=VECTOR('',#7075,10.);
#1737=VECTOR('',#7078,9.99999999999999);
#1738=VECTOR('',#7079,9.99999999999999);
#1739=VECTOR('',#7080,10.);
#1740=VECTOR('',#7083,10.);
#1741=VECTOR('',#7084,10.);
#1742=VECTOR('',#7085,10.);
#1743=VECTOR('',#7090,10.);
#1744=VECTOR('',#7097,10.);
#1745=VECTOR('',#7102,10.);
#1746=VECTOR('',#7103,10.);
#1747=VECTOR('',#7104,10.);
#1748=VECTOR('',#7105,10.);
#1749=VECTOR('',#7108,10.);
#1750=VECTOR('',#7109,10.);
#1751=VECTOR('',#7110,10.);
#1752=VECTOR('',#7113,9.99999999999999);
#1753=VECTOR('',#7114,10.);
#1754=VECTOR('',#7115,9.99999999999999);
#1755=VECTOR('',#7120,10.);
#1756=VECTOR('',#7127,10.);
#1757=VECTOR('',#7132,10.);
#1758=VECTOR('',#7133,10.);
#1759=VECTOR('',#7134,10.);
#1760=VECTOR('',#7135,10.);
#1761=VECTOR('',#7138,10.);
#1762=VECTOR('',#7139,10.);
#1763=VECTOR('',#7142,10.);
#1764=VECTOR('',#7143,10.);
#1765=VECTOR('',#7146,10.);
#1766=VECTOR('',#7147,10.);
#1767=VECTOR('',#7148,10.);
#1768=VECTOR('',#7149,10.);
#1769=VECTOR('',#7152,10.);
#1770=VECTOR('',#7153,10.);
#1771=VECTOR('',#7156,10.);
#1772=VECTOR('',#7157,10.);
#1773=VECTOR('',#7160,10.);
#1774=VECTOR('',#7161,10.);
#1775=VECTOR('',#7162,10.);
#1776=VECTOR('',#7163,10.);
#1777=VECTOR('',#7166,10.);
#1778=VECTOR('',#7167,10.);
#1779=VECTOR('',#7168,10.);
#1780=VECTOR('',#7171,10.);
#1781=VECTOR('',#7172,10.);
#1782=VECTOR('',#7177,10.);
#1783=VECTOR('',#7182,10.);
#1784=VECTOR('',#7183,10.);
#1785=VECTOR('',#7184,10.);
#1786=VECTOR('',#7185,10.);
#1787=VECTOR('',#7188,10.);
#1788=VECTOR('',#7189,10.);
#1789=VECTOR('',#7190,10.);
#1790=VECTOR('',#7193,10.);
#1791=VECTOR('',#7194,10.);
#1792=VECTOR('',#7199,10.);
#1793=VECTOR('',#7204,10.);
#1794=VECTOR('',#7205,10.);
#1795=VECTOR('',#7206,10.);
#1796=VECTOR('',#7207,10.);
#1797=VECTOR('',#7210,10.);
#1798=VECTOR('',#7211,10.);
#1799=VECTOR('',#7212,10.);
#1800=VECTOR('',#7215,10.);
#1801=VECTOR('',#7216,10.);
#1802=VECTOR('',#7217,10.);
#1803=VECTOR('',#7222,10.);
#1804=VECTOR('',#7229,10.);
#1805=VECTOR('',#7234,10.);
#1806=VECTOR('',#7235,10.);
#1807=VECTOR('',#7236,10.);
#1808=VECTOR('',#7237,10.);
#1809=VECTOR('',#7240,10.);
#1810=VECTOR('',#7241,10.);
#1811=VECTOR('',#7242,10.);
#1812=VECTOR('',#7245,10.);
#1813=VECTOR('',#7246,10.);
#1814=VECTOR('',#7251,10.);
#1815=VECTOR('',#7256,10.);
#1816=VECTOR('',#7257,10.);
#1817=VECTOR('',#7258,10.);
#1818=VECTOR('',#7259,10.);
#1819=VECTOR('',#7262,10.);
#1820=VECTOR('',#7263,10.);
#1821=VECTOR('',#7264,10.);
#1822=VECTOR('',#7267,10.);
#1823=VECTOR('',#7268,10.);
#1824=VECTOR('',#7273,10.);
#1825=VECTOR('',#7278,10.);
#1826=VECTOR('',#7279,10.);
#1827=VECTOR('',#7280,10.);
#1828=VECTOR('',#7281,10.);
#1829=VECTOR('',#7284,10.);
#1830=VECTOR('',#7285,10.);
#1831=VECTOR('',#7288,10.);
#1832=VECTOR('',#7289,10.);
#1833=VECTOR('',#7292,10.);
#1834=VECTOR('',#7293,10.);
#1835=VECTOR('',#7294,10.);
#1836=VECTOR('',#7295,10.);
#1837=VECTOR('',#7298,10.);
#1838=VECTOR('',#7299,10.);
#1839=VECTOR('',#7300,10.);
#1840=VECTOR('',#7303,10.);
#1841=VECTOR('',#7304,10.);
#1842=VECTOR('',#7305,10.);
#1843=VECTOR('',#7310,10.);
#1844=VECTOR('',#7317,10.);
#1845=VECTOR('',#7322,10.);
#1846=VECTOR('',#7323,10.);
#1847=VECTOR('',#7324,10.);
#1848=VECTOR('',#7325,10.);
#1849=VECTOR('',#7328,10.);
#1850=VECTOR('',#7329,10.);
#1851=VECTOR('',#7332,10.);
#1852=VECTOR('',#7333,10.);
#1853=VECTOR('',#7336,10.);
#1854=VECTOR('',#7337,10.);
#1855=VECTOR('',#7338,10.);
#1856=VECTOR('',#7339,10.);
#1857=VECTOR('',#7342,10.);
#1858=VECTOR('',#7343,10.);
#1859=VECTOR('',#7344,10.);
#1860=VECTOR('',#7347,10.);
#1861=VECTOR('',#7348,10.);
#1862=VECTOR('',#7349,10.);
#1863=VECTOR('',#7354,10.);
#1864=VECTOR('',#7361,10.);
#1865=VECTOR('',#7366,10.);
#1866=VECTOR('',#7367,10.);
#1867=VECTOR('',#7368,10.);
#1868=VECTOR('',#7369,10.);
#1869=VECTOR('',#7372,10.);
#1870=VECTOR('',#7373,10.);
#1871=VECTOR('',#7376,10.);
#1872=VECTOR('',#7377,10.);
#1873=VECTOR('',#7380,10.);
#1874=VECTOR('',#7381,10.);
#1875=VECTOR('',#7382,10.);
#1876=VECTOR('',#7383,10.);
#1877=VECTOR('',#7386,10.);
#1878=VECTOR('',#7387,10.);
#1879=VECTOR('',#7388,10.);
#1880=VECTOR('',#7391,10.);
#1881=VECTOR('',#7392,10.);
#1882=VECTOR('',#7393,10.);
#1883=VECTOR('',#7398,10.);
#1884=VECTOR('',#7405,10.);
#1885=VECTOR('',#7410,10.);
#1886=VECTOR('',#7411,10.);
#1887=VECTOR('',#7412,10.);
#1888=VECTOR('',#7413,10.);
#1889=VECTOR('',#7416,10.);
#1890=VECTOR('',#7417,10.);
#1891=VECTOR('',#7418,10.);
#1892=VECTOR('',#7421,10.);
#1893=VECTOR('',#7422,10.);
#1894=VECTOR('',#7427,10.);
#1895=VECTOR('',#7432,10.);
#1896=VECTOR('',#7433,10.);
#1897=VECTOR('',#7434,10.);
#1898=VECTOR('',#7435,10.);
#1899=VECTOR('',#7438,10.);
#1900=VECTOR('',#7439,10.);
#1901=VECTOR('',#7440,10.);
#1902=VECTOR('',#7443,10.);
#1903=VECTOR('',#7444,10.);
#1904=VECTOR('',#7449,10.);
#1905=VECTOR('',#7454,10.);
#1906=VECTOR('',#7455,10.);
#1907=VECTOR('',#7456,10.);
#1908=VECTOR('',#7457,10.);
#1909=VECTOR('',#7460,10.);
#1910=VECTOR('',#7461,10.);
#1911=VECTOR('',#7464,10.);
#1912=VECTOR('',#7465,10.);
#1913=VECTOR('',#7466,10.);
#1914=VECTOR('',#7471,10.);
#1915=VECTOR('',#7476,10.);
#1916=VECTOR('',#7477,10.);
#1917=VECTOR('',#7478,10.);
#1918=VECTOR('',#7479,10.);
#1919=VECTOR('',#7482,10.);
#1920=VECTOR('',#7483,10.);
#1921=VECTOR('',#7484,10.);
#1922=VECTOR('',#7487,10.);
#1923=VECTOR('',#7488,10.);
#1924=VECTOR('',#7489,10.);
#1925=VECTOR('',#7494,10.);
#1926=VECTOR('',#7501,10.);
#1927=VECTOR('',#7506,10.);
#1928=VECTOR('',#7507,10.);
#1929=VECTOR('',#7508,10.);
#1930=VECTOR('',#7509,10.);
#1931=VECTOR('',#7512,10.);
#1932=VECTOR('',#7513,10.);
#1933=VECTOR('',#7516,10.);
#1934=VECTOR('',#7517,10.);
#1935=VECTOR('',#7520,10.);
#1936=VECTOR('',#7521,10.);
#1937=VECTOR('',#7522,10.);
#1938=VECTOR('',#7523,10.);
#1939=VECTOR('',#7526,10.);
#1940=VECTOR('',#7527,10.);
#1941=VECTOR('',#7530,10.);
#1942=VECTOR('',#7531,10.);
#1943=VECTOR('',#7534,10.);
#1944=VECTOR('',#7535,10.);
#1945=VECTOR('',#7536,10.);
#1946=VECTOR('',#7537,10.);
#1947=VECTOR('',#7540,10.);
#1948=VECTOR('',#7541,10.);
#1949=VECTOR('',#7544,10.);
#1950=VECTOR('',#7545,10.);
#1951=VECTOR('',#7548,10.);
#1952=VECTOR('',#7549,10.);
#1953=VECTOR('',#7550,10.);
#1954=VECTOR('',#7551,10.);
#1955=VECTOR('',#7554,10.);
#1956=VECTOR('',#7555,10.);
#1957=VECTOR('',#7556,10.);
#1958=VECTOR('',#7557,10.);
#1959=VECTOR('',#7562,10.);
#1960=VECTOR('',#7569,10.);
#1961=VECTOR('',#7576,10.);
#1962=VECTOR('',#7583,10.);
#1963=VECTOR('',#7588,10.);
#1964=VECTOR('',#7589,10.);
#1965=VECTOR('',#7592,10.);
#1966=VECTOR('',#7593,10.);
#1967=VECTOR('',#7594,10.);
#1968=VECTOR('',#7595,10.);
#1969=VECTOR('',#7600,10.);
#1970=VECTOR('',#7607,10.);
#1971=VECTOR('',#7612,10.);
#1972=VECTOR('',#7613,10.);
#1973=VECTOR('',#7616,10.);
#1974=VECTOR('',#7617,10.);
#1975=VECTOR('',#7618,10.);
#1976=VECTOR('',#7619,10.);
#1977=VECTOR('',#7624,10.);
#1978=VECTOR('',#7631,10.);
#1979=VECTOR('',#7636,10.);
#1980=VECTOR('',#7637,10.);
#1981=VECTOR('',#7640,10.);
#1982=VECTOR('',#7641,10.);
#1983=VECTOR('',#7642,10.);
#1984=VECTOR('',#7643,10.);
#1985=VECTOR('',#7648,10.);
#1986=VECTOR('',#7655,10.);
#1987=VECTOR('',#7660,10.);
#1988=VECTOR('',#7661,10.);
#1989=VECTOR('',#7664,10.);
#1990=VECTOR('',#7665,10.);
#1991=VECTOR('',#7666,10.);
#1992=VECTOR('',#7667,10.);
#1993=VECTOR('',#7672,10.);
#1994=VECTOR('',#7679,10.);
#1995=VECTOR('',#7684,9.99999999999999);
#1996=VECTOR('',#7685,9.99999999999999);
#1997=VECTOR('',#7688,10.);
#1998=VECTOR('',#7689,10.);
#1999=VECTOR('',#7694,6.00000000000001);
#2181=CIRCLE('',#5953,25.5);
#2182=CIRCLE('',#5954,25.5);
#2183=CIRCLE('',#5956,25.5);
#2184=CIRCLE('',#5957,25.5);
#2185=CIRCLE('',#5962,25.5);
#2186=CIRCLE('',#5963,25.5);
#2187=CIRCLE('',#5968,25.5);
#2188=CIRCLE('',#5969,25.5);
#2189=CIRCLE('',#5974,25.5);
#2190=CIRCLE('',#5975,25.5);
#2191=CIRCLE('',#5980,25.5);
#2192=CIRCLE('',#5981,25.5);
#2193=CIRCLE('',#5986,25.5);
#2194=CIRCLE('',#5987,25.5);
#2195=CIRCLE('',#5989,25.5);
#2196=CIRCLE('',#5990,25.5);
#2197=CIRCLE('',#5998,25.5);
#2198=CIRCLE('',#5999,25.5);
#2199=CIRCLE('',#6004,25.5);
#2200=CIRCLE('',#6005,25.5);
#2201=CIRCLE('',#6007,25.5);
#2202=CIRCLE('',#6008,25.5);
#2203=CIRCLE('',#6013,25.5);
#2204=CIRCLE('',#6014,25.5);
#2205=CIRCLE('',#6016,25.5);
#2206=CIRCLE('',#6017,25.5);
#2207=CIRCLE('',#6028,25.5);
#2208=CIRCLE('',#6029,25.5);
#2209=CIRCLE('',#6034,25.5);
#2210=CIRCLE('',#6035,25.5);
#2211=CIRCLE('',#6040,25.5);
#2212=CIRCLE('',#6041,25.5);
#2213=CIRCLE('',#6043,25.5);
#2214=CIRCLE('',#6044,25.5);
#2215=CIRCLE('',#6049,25.5);
#2216=CIRCLE('',#6050,25.5);
#2217=CIRCLE('',#6055,25.5);
#2218=CIRCLE('',#6056,25.5);
#2219=CIRCLE('',#6064,25.5);
#2220=CIRCLE('',#6065,25.5);
#2221=CIRCLE('',#6067,25.5);
#2222=CIRCLE('',#6068,25.5);
#2223=CIRCLE('',#6076,25.5);
#2224=CIRCLE('',#6077,25.5);
#2225=CIRCLE('',#6079,25.5);
#2226=CIRCLE('',#6080,25.5);
#2227=CIRCLE('',#6088,25.5);
#2228=CIRCLE('',#6089,25.5);
#2229=CIRCLE('',#6091,25.5);
#2230=CIRCLE('',#6092,25.5);
#2231=CIRCLE('',#6097,25.5);
#2232=CIRCLE('',#6098,25.5);
#2233=CIRCLE('',#6103,25.5);
#2234=CIRCLE('',#6104,25.5);
#2235=CIRCLE('',#6109,25.5);
#2236=CIRCLE('',#6110,25.5);
#2237=CIRCLE('',#6115,25.5);
#2238=CIRCLE('',#6116,25.5);
#2239=CIRCLE('',#6118,25.5);
#2240=CIRCLE('',#6119,25.5);
#2241=CIRCLE('',#6132,22.);
#2242=CIRCLE('',#6133,22.);
#2243=CIRCLE('',#6135,22.);
#2244=CIRCLE('',#6136,22.);
#2245=CIRCLE('',#6138,7.00000000000001);
#2246=CIRCLE('',#6139,7.00000000000001);
#2247=CIRCLE('',#6141,7.00000000000001);
#2248=CIRCLE('',#6142,7.00000000000001);
#2249=CIRCLE('',#6146,22.);
#2250=CIRCLE('',#6147,22.);
#2251=CIRCLE('',#6149,7.00000000000001);
#2252=CIRCLE('',#6150,7.00000000000001);
#2253=CIRCLE('',#6154,22.);
#2254=CIRCLE('',#6155,22.);
#2255=CIRCLE('',#6157,7.00000000000001);
#2256=CIRCLE('',#6158,7.00000000000001);
#2257=CIRCLE('',#6162,22.);
#2258=CIRCLE('',#6163,22.);
#2259=CIRCLE('',#6165,7.00000000000001);
#2260=CIRCLE('',#6166,7.00000000000001);
#2261=CIRCLE('',#6170,22.);
#2262=CIRCLE('',#6171,22.);
#2263=CIRCLE('',#6173,7.00000000000001);
#2264=CIRCLE('',#6174,7.00000000000001);
#2265=CIRCLE('',#6178,6.00000000000001);
#2266=CIRCLE('',#6179,6.00000000000001);
#2480=VERTEX_POINT('',#8654);
#2481=VERTEX_POINT('',#8655);
#2482=VERTEX_POINT('',#8657);
#2483=VERTEX_POINT('',#8659);
#2484=VERTEX_POINT('',#8663);
#2485=VERTEX_POINT('',#8665);
#2486=VERTEX_POINT('',#8669);
#2487=VERTEX_POINT('',#8671);
#2488=VERTEX_POINT('',#8675);
#2489=VERTEX_POINT('',#8677);
#2490=VERTEX_POINT('',#8681);
#2491=VERTEX_POINT('',#8683);
#2492=VERTEX_POINT('',#8687);
#2493=VERTEX_POINT('',#8688);
#2494=VERTEX_POINT('',#8690);
#2495=VERTEX_POINT('',#8692);
#2496=VERTEX_POINT('',#8696);
#2497=VERTEX_POINT('',#8698);
#2498=VERTEX_POINT('',#8705);
#2499=VERTEX_POINT('',#8707);
#2500=VERTEX_POINT('',#8711);
#2501=VERTEX_POINT('',#8712);
#2502=VERTEX_POINT('',#8714);
#2503=VERTEX_POINT('',#8716);
#2504=VERTEX_POINT('',#8720);
#2505=VERTEX_POINT('',#8722);
#2506=VERTEX_POINT('',#8729);
#2507=VERTEX_POINT('',#8731);
#2508=VERTEX_POINT('',#8735);
#2509=VERTEX_POINT('',#8736);
#2510=VERTEX_POINT('',#8738);
#2511=VERTEX_POINT('',#8740);
#2512=VERTEX_POINT('',#8744);
#2513=VERTEX_POINT('',#8746);
#2514=VERTEX_POINT('',#8753);
#2515=VERTEX_POINT('',#8755);
#2516=VERTEX_POINT('',#8759);
#2517=VERTEX_POINT('',#8760);
#2518=VERTEX_POINT('',#8762);
#2519=VERTEX_POINT('',#8764);
#2520=VERTEX_POINT('',#8768);
#2521=VERTEX_POINT('',#8770);
#2522=VERTEX_POINT('',#8777);
#2523=VERTEX_POINT('',#8779);
#2524=VERTEX_POINT('',#8783);
#2525=VERTEX_POINT('',#8784);
#2526=VERTEX_POINT('',#8786);
#2527=VERTEX_POINT('',#8788);
#2528=VERTEX_POINT('',#8792);
#2529=VERTEX_POINT('',#8794);
#2530=VERTEX_POINT('',#8798);
#2531=VERTEX_POINT('',#8800);
#2532=VERTEX_POINT('',#8804);
#2533=VERTEX_POINT('',#8806);
#2534=VERTEX_POINT('',#8810);
#2535=VERTEX_POINT('',#8812);
#2536=VERTEX_POINT('',#8816);
#2537=VERTEX_POINT('',#8817);
#2538=VERTEX_POINT('',#8819);
#2539=VERTEX_POINT('',#8821);
#2540=VERTEX_POINT('',#8831);
#2541=VERTEX_POINT('',#8832);
#2542=VERTEX_POINT('',#8834);
#2543=VERTEX_POINT('',#8836);
#2544=VERTEX_POINT('',#8840);
#2545=VERTEX_POINT('',#8842);
#2546=VERTEX_POINT('',#8849);
#2547=VERTEX_POINT('',#8851);
#2548=VERTEX_POINT('',#8855);
#2549=VERTEX_POINT('',#8856);
#2550=VERTEX_POINT('',#8858);
#2551=VERTEX_POINT('',#8860);
#2552=VERTEX_POINT('',#8864);
#2553=VERTEX_POINT('',#8866);
#2554=VERTEX_POINT('',#8870);
#2555=VERTEX_POINT('',#8872);
#2556=VERTEX_POINT('',#8876);
#2557=VERTEX_POINT('',#8878);
#2558=VERTEX_POINT('',#8882);
#2559=VERTEX_POINT('',#8884);
#2560=VERTEX_POINT('',#8888);
#2561=VERTEX_POINT('',#8889);
#2562=VERTEX_POINT('',#8891);
#2563=VERTEX_POINT('',#8893);
#2564=VERTEX_POINT('',#8897);
#2565=VERTEX_POINT('',#8899);
#2566=VERTEX_POINT('',#8903);
#2567=VERTEX_POINT('',#8905);
#2568=VERTEX_POINT('',#8909);
#2569=VERTEX_POINT('',#8911);
#2570=VERTEX_POINT('',#8915);
#2571=VERTEX_POINT('',#8917);
#2572=VERTEX_POINT('',#8921);
#2573=VERTEX_POINT('',#8922);
#2574=VERTEX_POINT('',#8924);
#2575=VERTEX_POINT('',#8926);
#2576=VERTEX_POINT('',#8936);
#2577=VERTEX_POINT('',#8937);
#2578=VERTEX_POINT('',#8939);
#2579=VERTEX_POINT('',#8941);
#2580=VERTEX_POINT('',#8951);
#2581=VERTEX_POINT('',#8952);
#2582=VERTEX_POINT('',#8954);
#2583=VERTEX_POINT('',#8956);
#2584=VERTEX_POINT('',#8960);
#2585=VERTEX_POINT('',#8962);
#2586=VERTEX_POINT('',#8969);
#2587=VERTEX_POINT('',#8971);
#2588=VERTEX_POINT('',#8975);
#2589=VERTEX_POINT('',#8976);
#2590=VERTEX_POINT('',#8978);
#2591=VERTEX_POINT('',#8980);
#2592=VERTEX_POINT('',#8984);
#2593=VERTEX_POINT('',#8986);
#2594=VERTEX_POINT('',#8993);
#2595=VERTEX_POINT('',#8995);
#2596=VERTEX_POINT('',#8999);
#2597=VERTEX_POINT('',#9000);
#2598=VERTEX_POINT('',#9002);
#2599=VERTEX_POINT('',#9004);
#2600=VERTEX_POINT('',#9008);
#2601=VERTEX_POINT('',#9010);
#2602=VERTEX_POINT('',#9014);
#2603=VERTEX_POINT('',#9016);
#2604=VERTEX_POINT('',#9020);
#2605=VERTEX_POINT('',#9022);
#2606=VERTEX_POINT('',#9026);
#2607=VERTEX_POINT('',#9028);
#2608=VERTEX_POINT('',#9032);
#2609=VERTEX_POINT('',#9033);
#2610=VERTEX_POINT('',#9035);
#2611=VERTEX_POINT('',#9037);
#2612=VERTEX_POINT('',#9041);
#2613=VERTEX_POINT('',#9043);
#2614=VERTEX_POINT('',#9050);
#2615=VERTEX_POINT('',#9052);
#2616=VERTEX_POINT('',#9056);
#2617=VERTEX_POINT('',#9057);
#2618=VERTEX_POINT('',#9059);
#2619=VERTEX_POINT('',#9061);
#2620=VERTEX_POINT('',#9065);
#2621=VERTEX_POINT('',#9067);
#2622=VERTEX_POINT('',#9074);
#2623=VERTEX_POINT('',#9076);
#2624=VERTEX_POINT('',#9080);
#2625=VERTEX_POINT('',#9081);
#2626=VERTEX_POINT('',#9083);
#2627=VERTEX_POINT('',#9085);
#2628=VERTEX_POINT('',#9095);
#2629=VERTEX_POINT('',#9096);
#2630=VERTEX_POINT('',#9098);
#2631=VERTEX_POINT('',#9100);
#2632=VERTEX_POINT('',#9104);
#2633=VERTEX_POINT('',#9106);
#2634=VERTEX_POINT('',#9110);
#2635=VERTEX_POINT('',#9112);
#2636=VERTEX_POINT('',#9116);
#2637=VERTEX_POINT('',#9118);
#2638=VERTEX_POINT('',#9122);
#2639=VERTEX_POINT('',#9124);
#2640=VERTEX_POINT('',#9128);
#2641=VERTEX_POINT('',#9129);
#2642=VERTEX_POINT('',#9131);
#2643=VERTEX_POINT('',#9133);
#2644=VERTEX_POINT('',#9143);
#2645=VERTEX_POINT('',#9144);
#2646=VERTEX_POINT('',#9146);
#2647=VERTEX_POINT('',#9148);
#2648=VERTEX_POINT('',#9152);
#2649=VERTEX_POINT('',#9154);
#2650=VERTEX_POINT('',#9158);
#2651=VERTEX_POINT('',#9160);
#2652=VERTEX_POINT('',#9164);
#2653=VERTEX_POINT('',#9166);
#2654=VERTEX_POINT('',#9170);
#2655=VERTEX_POINT('',#9172);
#2656=VERTEX_POINT('',#9176);
#2657=VERTEX_POINT('',#9177);
#2658=VERTEX_POINT('',#9179);
#2659=VERTEX_POINT('',#9181);
#2660=VERTEX_POINT('',#9191);
#2661=VERTEX_POINT('',#9192);
#2662=VERTEX_POINT('',#9194);
#2663=VERTEX_POINT('',#9196);
#2664=VERTEX_POINT('',#9200);
#2665=VERTEX_POINT('',#9202);
#2666=VERTEX_POINT('',#9206);
#2667=VERTEX_POINT('',#9208);
#2668=VERTEX_POINT('',#9212);
#2669=VERTEX_POINT('',#9214);
#2670=VERTEX_POINT('',#9218);
#2671=VERTEX_POINT('',#9220);
#2672=VERTEX_POINT('',#9224);
#2673=VERTEX_POINT('',#9225);
#2674=VERTEX_POINT('',#9227);
#2675=VERTEX_POINT('',#9229);
#2676=VERTEX_POINT('',#9233);
#2677=VERTEX_POINT('',#9235);
#2678=VERTEX_POINT('',#9242);
#2679=VERTEX_POINT('',#9244);
#2680=VERTEX_POINT('',#9248);
#2681=VERTEX_POINT('',#9249);
#2682=VERTEX_POINT('',#9251);
#2683=VERTEX_POINT('',#9253);
#2684=VERTEX_POINT('',#9257);
#2685=VERTEX_POINT('',#9259);
#2686=VERTEX_POINT('',#9266);
#2687=VERTEX_POINT('',#9268);
#2688=VERTEX_POINT('',#9272);
#2689=VERTEX_POINT('',#9273);
#2690=VERTEX_POINT('',#9275);
#2691=VERTEX_POINT('',#9277);
#2692=VERTEX_POINT('',#9284);
#2693=VERTEX_POINT('',#9286);
#2694=VERTEX_POINT('',#9290);
#2695=VERTEX_POINT('',#9292);
#2696=VERTEX_POINT('',#9296);
#2697=VERTEX_POINT('',#9297);
#2698=VERTEX_POINT('',#9299);
#2699=VERTEX_POINT('',#9301);
#2700=VERTEX_POINT('',#9305);
#2701=VERTEX_POINT('',#9307);
#2702=VERTEX_POINT('',#9311);
#2703=VERTEX_POINT('',#9313);
#2704=VERTEX_POINT('',#9317);
#2705=VERTEX_POINT('',#9319);
#2706=VERTEX_POINT('',#9323);
#2707=VERTEX_POINT('',#9325);
#2708=VERTEX_POINT('',#9329);
#2709=VERTEX_POINT('',#9330);
#2710=VERTEX_POINT('',#9332);
#2711=VERTEX_POINT('',#9334);
#2712=VERTEX_POINT('',#9344);
#2713=VERTEX_POINT('',#9345);
#2714=VERTEX_POINT('',#9347);
#2715=VERTEX_POINT('',#9349);
#2716=VERTEX_POINT('',#9359);
#2717=VERTEX_POINT('',#9360);
#2718=VERTEX_POINT('',#9362);
#2719=VERTEX_POINT('',#9364);
#2720=VERTEX_POINT('',#9374);
#2721=VERTEX_POINT('',#9375);
#2722=VERTEX_POINT('',#9377);
#2723=VERTEX_POINT('',#9379);
#2724=VERTEX_POINT('',#9383);
#2725=VERTEX_POINT('',#9384);
#2726=VERTEX_POINT('',#9386);
#2727=VERTEX_POINT('',#9388);
#2728=VERTEX_POINT('',#9392);
#2729=VERTEX_POINT('',#9394);
#2730=VERTEX_POINT('',#9398);
#2731=VERTEX_POINT('',#9400);
#2732=VERTEX_POINT('',#9404);
#2733=VERTEX_POINT('',#9406);
#2734=VERTEX_POINT('',#9410);
#2735=VERTEX_POINT('',#9412);
#2736=VERTEX_POINT('',#9419);
#2737=VERTEX_POINT('',#9420);
#2738=VERTEX_POINT('',#9422);
#2739=VERTEX_POINT('',#9424);
#2740=VERTEX_POINT('',#9428);
#2741=VERTEX_POINT('',#9430);
#2742=VERTEX_POINT('',#9434);
#2743=VERTEX_POINT('',#9436);
#2744=VERTEX_POINT('',#9443);
#2745=VERTEX_POINT('',#9444);
#2746=VERTEX_POINT('',#9446);
#2747=VERTEX_POINT('',#9448);
#2748=VERTEX_POINT('',#9452);
#2749=VERTEX_POINT('',#9454);
#2750=VERTEX_POINT('',#9458);
#2751=VERTEX_POINT('',#9460);
#2752=VERTEX_POINT('',#9467);
#2753=VERTEX_POINT('',#9468);
#2754=VERTEX_POINT('',#9470);
#2755=VERTEX_POINT('',#9472);
#2756=VERTEX_POINT('',#9476);
#2757=VERTEX_POINT('',#9478);
#2758=VERTEX_POINT('',#9482);
#2759=VERTEX_POINT('',#9484);
#2760=VERTEX_POINT('',#9491);
#2761=VERTEX_POINT('',#9492);
#2762=VERTEX_POINT('',#9494);
#2763=VERTEX_POINT('',#9496);
#2764=VERTEX_POINT('',#9500);
#2765=VERTEX_POINT('',#9502);
#2766=VERTEX_POINT('',#9506);
#2767=VERTEX_POINT('',#9508);
#2768=VERTEX_POINT('',#9518);
#2769=VERTEX_POINT('',#9520);
#3053=EDGE_CURVE('',#2480,#2481,#1187,.T.);
#3054=EDGE_CURVE('',#2480,#2482,#1188,.T.);
#3055=EDGE_CURVE('',#2483,#2482,#1189,.T.);
#3056=EDGE_CURVE('',#2481,#2483,#1190,.T.);
#3057=EDGE_CURVE('',#2481,#2484,#1191,.T.);
#3058=EDGE_CURVE('',#2485,#2483,#1192,.T.);
#3059=EDGE_CURVE('',#2484,#2485,#1193,.T.);
#3060=EDGE_CURVE('',#2480,#2486,#1194,.T.);
#3061=EDGE_CURVE('',#2487,#2486,#1195,.T.);
#3062=EDGE_CURVE('',#2482,#2487,#1196,.T.);
#3063=EDGE_CURVE('',#2488,#2485,#2181,.T.);
#3064=EDGE_CURVE('',#2488,#2489,#1197,.T.);
#3065=EDGE_CURVE('',#2489,#2484,#2182,.T.);
#3066=EDGE_CURVE('',#2486,#2490,#2183,.T.);
#3067=EDGE_CURVE('',#2490,#2491,#1198,.T.);
#3068=EDGE_CURVE('',#2487,#2491,#2184,.T.);
#3069=EDGE_CURVE('',#2492,#2493,#1199,.T.);
#3070=EDGE_CURVE('',#2492,#2494,#1200,.T.);
#3071=EDGE_CURVE('',#2495,#2494,#1201,.T.);
#3072=EDGE_CURVE('',#2493,#2495,#1202,.T.);
#3073=EDGE_CURVE('',#2493,#2496,#1203,.T.);
#3074=EDGE_CURVE('',#2497,#2495,#1204,.T.);
#3075=EDGE_CURVE('',#2496,#2497,#1205,.T.);
#3076=EDGE_CURVE('',#2492,#2489,#1206,.T.);
#3077=EDGE_CURVE('',#2494,#2488,#1207,.T.);
#3078=EDGE_CURVE('',#2498,#2497,#2185,.T.);
#3079=EDGE_CURVE('',#2498,#2499,#1208,.T.);
#3080=EDGE_CURVE('',#2499,#2496,#2186,.T.);
#3081=EDGE_CURVE('',#2500,#2501,#1209,.T.);
#3082=EDGE_CURVE('',#2500,#2502,#1210,.T.);
#3083=EDGE_CURVE('',#2503,#2502,#1211,.T.);
#3084=EDGE_CURVE('',#2501,#2503,#1212,.T.);
#3085=EDGE_CURVE('',#2501,#2504,#1213,.T.);
#3086=EDGE_CURVE('',#2505,#2503,#1214,.T.);
#3087=EDGE_CURVE('',#2504,#2505,#1215,.T.);
#3088=EDGE_CURVE('',#2500,#2499,#1216,.T.);
#3089=EDGE_CURVE('',#2502,#2498,#1217,.T.);
#3090=EDGE_CURVE('',#2506,#2505,#2187,.T.);
#3091=EDGE_CURVE('',#2506,#2507,#1218,.T.);
#3092=EDGE_CURVE('',#2507,#2504,#2188,.T.);
#3093=EDGE_CURVE('',#2508,#2509,#1219,.T.);
#3094=EDGE_CURVE('',#2508,#2510,#1220,.T.);
#3095=EDGE_CURVE('',#2511,#2510,#1221,.T.);
#3096=EDGE_CURVE('',#2509,#2511,#1222,.T.);
#3097=EDGE_CURVE('',#2509,#2512,#1223,.T.);
#3098=EDGE_CURVE('',#2513,#2511,#1224,.T.);
#3099=EDGE_CURVE('',#2512,#2513,#1225,.T.);
#3100=EDGE_CURVE('',#2508,#2507,#1226,.T.);
#3101=EDGE_CURVE('',#2510,#2506,#1227,.T.);
#3102=EDGE_CURVE('',#2514,#2513,#2189,.T.);
#3103=EDGE_CURVE('',#2514,#2515,#1228,.T.);
#3104=EDGE_CURVE('',#2515,#2512,#2190,.T.);
#3105=EDGE_CURVE('',#2516,#2517,#1229,.T.);
#3106=EDGE_CURVE('',#2516,#2518,#1230,.T.);
#3107=EDGE_CURVE('',#2519,#2518,#1231,.T.);
#3108=EDGE_CURVE('',#2517,#2519,#1232,.T.);
#3109=EDGE_CURVE('',#2517,#2520,#1233,.T.);
#3110=EDGE_CURVE('',#2521,#2519,#1234,.T.);
#3111=EDGE_CURVE('',#2520,#2521,#1235,.T.);
#3112=EDGE_CURVE('',#2516,#2515,#1236,.T.);
#3113=EDGE_CURVE('',#2518,#2514,#1237,.T.);
#3114=EDGE_CURVE('',#2522,#2521,#2191,.T.);
#3115=EDGE_CURVE('',#2522,#2523,#1238,.T.);
#3116=EDGE_CURVE('',#2523,#2520,#2192,.T.);
#3117=EDGE_CURVE('',#2524,#2525,#1239,.T.);
#3118=EDGE_CURVE('',#2524,#2526,#1240,.T.);
#3119=EDGE_CURVE('',#2527,#2526,#1241,.T.);
#3120=EDGE_CURVE('',#2525,#2527,#1242,.T.);
#3121=EDGE_CURVE('',#2525,#2528,#1243,.T.);
#3122=EDGE_CURVE('',#2529,#2527,#1244,.T.);
#3123=EDGE_CURVE('',#2528,#2529,#1245,.T.);
#3124=EDGE_CURVE('',#2524,#2530,#1246,.T.);
#3125=EDGE_CURVE('',#2531,#2530,#1247,.T.);
#3126=EDGE_CURVE('',#2526,#2531,#1248,.T.);
#3127=EDGE_CURVE('',#2532,#2529,#2193,.T.);
#3128=EDGE_CURVE('',#2532,#2533,#1249,.T.);
#3129=EDGE_CURVE('',#2533,#2528,#2194,.T.);
#3130=EDGE_CURVE('',#2530,#2534,#2195,.T.);
#3131=EDGE_CURVE('',#2534,#2535,#1250,.T.);
#3132=EDGE_CURVE('',#2531,#2535,#2196,.T.);
#3133=EDGE_CURVE('',#2536,#2537,#1251,.T.);
#3134=EDGE_CURVE('',#2536,#2538,#1252,.T.);
#3135=EDGE_CURVE('',#2539,#2538,#1253,.T.);
#3136=EDGE_CURVE('',#2537,#2539,#1254,.T.);
#3137=EDGE_CURVE('',#2537,#2534,#1255,.T.);
#3138=EDGE_CURVE('',#2535,#2539,#1256,.T.);
#3139=EDGE_CURVE('',#2536,#2523,#1257,.T.);
#3140=EDGE_CURVE('',#2538,#2522,#1258,.T.);
#3141=EDGE_CURVE('',#2540,#2541,#1259,.T.);
#3142=EDGE_CURVE('',#2540,#2542,#1260,.T.);
#3143=EDGE_CURVE('',#2543,#2542,#1261,.T.);
#3144=EDGE_CURVE('',#2541,#2543,#1262,.T.);
#3145=EDGE_CURVE('',#2541,#2544,#1263,.T.);
#3146=EDGE_CURVE('',#2545,#2543,#1264,.T.);
#3147=EDGE_CURVE('',#2544,#2545,#1265,.T.);
#3148=EDGE_CURVE('',#2540,#2533,#1266,.T.);
#3149=EDGE_CURVE('',#2542,#2532,#1267,.T.);
#3150=EDGE_CURVE('',#2546,#2545,#2197,.T.);
#3151=EDGE_CURVE('',#2546,#2547,#1268,.T.);
#3152=EDGE_CURVE('',#2547,#2544,#2198,.T.);
#3153=EDGE_CURVE('',#2548,#2549,#1269,.T.);
#3154=EDGE_CURVE('',#2548,#2550,#1270,.T.);
#3155=EDGE_CURVE('',#2551,#2550,#1271,.T.);
#3156=EDGE_CURVE('',#2549,#2551,#1272,.T.);
#3157=EDGE_CURVE('',#2549,#2552,#1273,.T.);
#3158=EDGE_CURVE('',#2553,#2551,#1274,.T.);
#3159=EDGE_CURVE('',#2552,#2553,#1275,.T.);
#3160=EDGE_CURVE('',#2548,#2554,#1276,.T.);
#3161=EDGE_CURVE('',#2555,#2554,#1277,.T.);
#3162=EDGE_CURVE('',#2550,#2555,#1278,.T.);
#3163=EDGE_CURVE('',#2556,#2553,#2199,.T.);
#3164=EDGE_CURVE('',#2556,#2557,#1279,.T.);
#3165=EDGE_CURVE('',#2557,#2552,#2200,.T.);
#3166=EDGE_CURVE('',#2554,#2558,#2201,.T.);
#3167=EDGE_CURVE('',#2558,#2559,#1280,.T.);
#3168=EDGE_CURVE('',#2555,#2559,#2202,.T.);
#3169=EDGE_CURVE('',#2560,#2561,#1281,.T.);
#3170=EDGE_CURVE('',#2560,#2562,#1282,.T.);
#3171=EDGE_CURVE('',#2563,#2562,#1283,.T.);
#3172=EDGE_CURVE('',#2561,#2563,#1284,.T.);
#3173=EDGE_CURVE('',#2561,#2564,#1285,.T.);
#3174=EDGE_CURVE('',#2565,#2563,#1286,.T.);
#3175=EDGE_CURVE('',#2564,#2565,#1287,.T.);
#3176=EDGE_CURVE('',#2560,#2566,#1288,.T.);
#3177=EDGE_CURVE('',#2567,#2566,#1289,.T.);
#3178=EDGE_CURVE('',#2562,#2567,#1290,.T.);
#3179=EDGE_CURVE('',#2568,#2565,#2203,.T.);
#3180=EDGE_CURVE('',#2568,#2569,#1291,.T.);
#3181=EDGE_CURVE('',#2569,#2564,#2204,.T.);
#3182=EDGE_CURVE('',#2566,#2570,#2205,.T.);
#3183=EDGE_CURVE('',#2570,#2571,#1292,.T.);
#3184=EDGE_CURVE('',#2567,#2571,#2206,.T.);
#3185=EDGE_CURVE('',#2572,#2573,#1293,.T.);
#3186=EDGE_CURVE('',#2572,#2574,#1294,.T.);
#3187=EDGE_CURVE('',#2575,#2574,#1295,.T.);
#3188=EDGE_CURVE('',#2573,#2575,#1296,.T.);
#3189=EDGE_CURVE('',#2573,#2570,#1297,.T.);
#3190=EDGE_CURVE('',#2571,#2575,#1298,.T.);
#3191=EDGE_CURVE('',#2572,#2557,#1299,.T.);
#3192=EDGE_CURVE('',#2574,#2556,#1300,.T.);
#3193=EDGE_CURVE('',#2576,#2577,#1301,.T.);
#3194=EDGE_CURVE('',#2576,#2578,#1302,.T.);
#3195=EDGE_CURVE('',#2579,#2578,#1303,.T.);
#3196=EDGE_CURVE('',#2577,#2579,#1304,.T.);
#3197=EDGE_CURVE('',#2577,#2558,#1305,.T.);
#3198=EDGE_CURVE('',#2559,#2579,#1306,.T.);
#3199=EDGE_CURVE('',#2576,#2547,#1307,.T.);
#3200=EDGE_CURVE('',#2578,#2546,#1308,.T.);
#3201=EDGE_CURVE('',#2580,#2581,#1309,.T.);
#3202=EDGE_CURVE('',#2580,#2582,#1310,.T.);
#3203=EDGE_CURVE('',#2583,#2582,#1311,.T.);
#3204=EDGE_CURVE('',#2581,#2583,#1312,.T.);
#3205=EDGE_CURVE('',#2581,#2584,#1313,.T.);
#3206=EDGE_CURVE('',#2585,#2583,#1314,.T.);
#3207=EDGE_CURVE('',#2584,#2585,#1315,.T.);
#3208=EDGE_CURVE('',#2580,#2569,#1316,.T.);
#3209=EDGE_CURVE('',#2582,#2568,#1317,.T.);
#3210=EDGE_CURVE('',#2586,#2585,#2207,.T.);
#3211=EDGE_CURVE('',#2586,#2587,#1318,.T.);
#3212=EDGE_CURVE('',#2587,#2584,#2208,.T.);
#3213=EDGE_CURVE('',#2588,#2589,#1319,.T.);
#3214=EDGE_CURVE('',#2588,#2590,#1320,.T.);
#3215=EDGE_CURVE('',#2591,#2590,#1321,.T.);
#3216=EDGE_CURVE('',#2589,#2591,#1322,.T.);
#3217=EDGE_CURVE('',#2589,#2592,#1323,.T.);
#3218=EDGE_CURVE('',#2593,#2591,#1324,.T.);
#3219=EDGE_CURVE('',#2592,#2593,#1325,.T.);
#3220=EDGE_CURVE('',#2588,#2587,#1326,.T.);
#3221=EDGE_CURVE('',#2590,#2586,#1327,.T.);
#3222=EDGE_CURVE('',#2594,#2593,#2209,.T.);
#3223=EDGE_CURVE('',#2594,#2595,#1328,.T.);
#3224=EDGE_CURVE('',#2595,#2592,#2210,.T.);
#3225=EDGE_CURVE('',#2596,#2597,#1329,.T.);
#3226=EDGE_CURVE('',#2596,#2598,#1330,.T.);
#3227=EDGE_CURVE('',#2599,#2598,#1331,.T.);
#3228=EDGE_CURVE('',#2597,#2599,#1332,.T.);
#3229=EDGE_CURVE('',#2597,#2600,#1333,.T.);
#3230=EDGE_CURVE('',#2601,#2599,#1334,.T.);
#3231=EDGE_CURVE('',#2600,#2601,#1335,.T.);
#3232=EDGE_CURVE('',#2596,#2602,#1336,.T.);
#3233=EDGE_CURVE('',#2603,#2602,#1337,.T.);
#3234=EDGE_CURVE('',#2598,#2603,#1338,.T.);
#3235=EDGE_CURVE('',#2604,#2601,#2211,.T.);
#3236=EDGE_CURVE('',#2604,#2605,#1339,.T.);
#3237=EDGE_CURVE('',#2605,#2600,#2212,.T.);
#3238=EDGE_CURVE('',#2602,#2606,#2213,.T.);
#3239=EDGE_CURVE('',#2606,#2607,#1340,.T.);
#3240=EDGE_CURVE('',#2603,#2607,#2214,.T.);
#3241=EDGE_CURVE('',#2608,#2609,#1341,.T.);
#3242=EDGE_CURVE('',#2608,#2610,#1342,.T.);
#3243=EDGE_CURVE('',#2611,#2610,#1343,.T.);
#3244=EDGE_CURVE('',#2609,#2611,#1344,.T.);
#3245=EDGE_CURVE('',#2609,#2612,#1345,.T.);
#3246=EDGE_CURVE('',#2613,#2611,#1346,.T.);
#3247=EDGE_CURVE('',#2612,#2613,#1347,.T.);
#3248=EDGE_CURVE('',#2608,#2595,#1348,.T.);
#3249=EDGE_CURVE('',#2610,#2594,#1349,.T.);
#3250=EDGE_CURVE('',#2614,#2613,#2215,.T.);
#3251=EDGE_CURVE('',#2614,#2615,#1350,.T.);
#3252=EDGE_CURVE('',#2615,#2612,#2216,.T.);
#3253=EDGE_CURVE('',#2616,#2617,#1351,.T.);
#3254=EDGE_CURVE('',#2616,#2618,#1352,.T.);
#3255=EDGE_CURVE('',#2619,#2618,#1353,.T.);
#3256=EDGE_CURVE('',#2617,#2619,#1354,.T.);
#3257=EDGE_CURVE('',#2617,#2620,#1355,.T.);
#3258=EDGE_CURVE('',#2621,#2619,#1356,.T.);
#3259=EDGE_CURVE('',#2620,#2621,#1357,.T.);
#3260=EDGE_CURVE('',#2616,#2615,#1358,.T.);
#3261=EDGE_CURVE('',#2618,#2614,#1359,.T.);
#3262=EDGE_CURVE('',#2622,#2621,#2217,.T.);
#3263=EDGE_CURVE('',#2622,#2623,#1360,.T.);
#3264=EDGE_CURVE('',#2623,#2620,#2218,.T.);
#3265=EDGE_CURVE('',#2624,#2625,#1361,.T.);
#3266=EDGE_CURVE('',#2624,#2626,#1362,.T.);
#3267=EDGE_CURVE('',#2627,#2626,#1363,.T.);
#3268=EDGE_CURVE('',#2625,#2627,#1364,.T.);
#3269=EDGE_CURVE('',#2625,#2606,#1365,.T.);
#3270=EDGE_CURVE('',#2607,#2627,#1366,.T.);
#3271=EDGE_CURVE('',#2624,#2623,#1367,.T.);
#3272=EDGE_CURVE('',#2626,#2622,#1368,.T.);
#3273=EDGE_CURVE('',#2628,#2629,#1369,.T.);
#3274=EDGE_CURVE('',#2628,#2630,#1370,.T.);
#3275=EDGE_CURVE('',#2631,#2630,#1371,.T.);
#3276=EDGE_CURVE('',#2629,#2631,#1372,.T.);
#3277=EDGE_CURVE('',#2629,#2632,#1373,.T.);
#3278=EDGE_CURVE('',#2633,#2631,#1374,.T.);
#3279=EDGE_CURVE('',#2632,#2633,#1375,.T.);
#3280=EDGE_CURVE('',#2628,#2634,#1376,.T.);
#3281=EDGE_CURVE('',#2635,#2634,#1377,.T.);
#3282=EDGE_CURVE('',#2630,#2635,#1378,.T.);
#3283=EDGE_CURVE('',#2636,#2633,#2219,.T.);
#3284=EDGE_CURVE('',#2636,#2637,#1379,.T.);
#3285=EDGE_CURVE('',#2637,#2632,#2220,.T.);
#3286=EDGE_CURVE('',#2634,#2638,#2221,.T.);
#3287=EDGE_CURVE('',#2638,#2639,#1380,.T.);
#3288=EDGE_CURVE('',#2635,#2639,#2222,.T.);
#3289=EDGE_CURVE('',#2640,#2641,#1381,.T.);
#3290=EDGE_CURVE('',#2640,#2642,#1382,.T.);
#3291=EDGE_CURVE('',#2643,#2642,#1383,.T.);
#3292=EDGE_CURVE('',#2641,#2643,#1384,.T.);
#3293=EDGE_CURVE('',#2641,#2638,#1385,.T.);
#3294=EDGE_CURVE('',#2639,#2643,#1386,.T.);
#3295=EDGE_CURVE('',#2640,#2605,#1387,.T.);
#3296=EDGE_CURVE('',#2642,#2604,#1388,.T.);
#3297=EDGE_CURVE('',#2644,#2645,#1389,.T.);
#3298=EDGE_CURVE('',#2644,#2646,#1390,.T.);
#3299=EDGE_CURVE('',#2647,#2646,#1391,.T.);
#3300=EDGE_CURVE('',#2645,#2647,#1392,.T.);
#3301=EDGE_CURVE('',#2645,#2648,#1393,.T.);
#3302=EDGE_CURVE('',#2649,#2647,#1394,.T.);
#3303=EDGE_CURVE('',#2648,#2649,#1395,.T.);
#3304=EDGE_CURVE('',#2644,#2650,#1396,.T.);
#3305=EDGE_CURVE('',#2651,#2650,#1397,.T.);
#3306=EDGE_CURVE('',#2646,#2651,#1398,.T.);
#3307=EDGE_CURVE('',#2652,#2649,#2223,.T.);
#3308=EDGE_CURVE('',#2652,#2653,#1399,.T.);
#3309=EDGE_CURVE('',#2653,#2648,#2224,.T.);
#3310=EDGE_CURVE('',#2650,#2654,#2225,.T.);
#3311=EDGE_CURVE('',#2654,#2655,#1400,.T.);
#3312=EDGE_CURVE('',#2651,#2655,#2226,.T.);
#3313=EDGE_CURVE('',#2656,#2657,#1401,.T.);
#3314=EDGE_CURVE('',#2656,#2658,#1402,.T.);
#3315=EDGE_CURVE('',#2659,#2658,#1403,.T.);
#3316=EDGE_CURVE('',#2657,#2659,#1404,.T.);
#3317=EDGE_CURVE('',#2657,#2490,#1405,.T.);
#3318=EDGE_CURVE('',#2491,#2659,#1406,.T.);
#3319=EDGE_CURVE('',#2656,#2653,#1407,.T.);
#3320=EDGE_CURVE('',#2658,#2652,#1408,.T.);
#3321=EDGE_CURVE('',#2660,#2661,#1409,.T.);
#3322=EDGE_CURVE('',#2660,#2662,#1410,.T.);
#3323=EDGE_CURVE('',#2663,#2662,#1411,.T.);
#3324=EDGE_CURVE('',#2661,#2663,#1412,.T.);
#3325=EDGE_CURVE('',#2661,#2664,#1413,.T.);
#3326=EDGE_CURVE('',#2665,#2663,#1414,.T.);
#3327=EDGE_CURVE('',#2664,#2665,#1415,.T.);
#3328=EDGE_CURVE('',#2660,#2666,#1416,.T.);
#3329=EDGE_CURVE('',#2667,#2666,#1417,.T.);
#3330=EDGE_CURVE('',#2662,#2667,#1418,.T.);
#3331=EDGE_CURVE('',#2668,#2665,#2227,.T.);
#3332=EDGE_CURVE('',#2668,#2669,#1419,.T.);
#3333=EDGE_CURVE('',#2669,#2664,#2228,.T.);
#3334=EDGE_CURVE('',#2666,#2670,#2229,.T.);
#3335=EDGE_CURVE('',#2670,#2671,#1420,.T.);
#3336=EDGE_CURVE('',#2667,#2671,#2230,.T.);
#3337=EDGE_CURVE('',#2672,#2673,#1421,.T.);
#3338=EDGE_CURVE('',#2672,#2674,#1422,.T.);
#3339=EDGE_CURVE('',#2675,#2674,#1423,.T.);
#3340=EDGE_CURVE('',#2673,#2675,#1424,.T.);
#3341=EDGE_CURVE('',#2673,#2676,#1425,.T.);
#3342=EDGE_CURVE('',#2677,#2675,#1426,.T.);
#3343=EDGE_CURVE('',#2676,#2677,#1427,.T.);
#3344=EDGE_CURVE('',#2672,#2669,#1428,.T.);
#3345=EDGE_CURVE('',#2674,#2668,#1429,.T.);
#3346=EDGE_CURVE('',#2678,#2677,#2231,.T.);
#3347=EDGE_CURVE('',#2678,#2679,#1430,.T.);
#3348=EDGE_CURVE('',#2679,#2676,#2232,.T.);
#3349=EDGE_CURVE('',#2680,#2681,#1431,.T.);
#3350=EDGE_CURVE('',#2680,#2682,#1432,.T.);
#3351=EDGE_CURVE('',#2683,#2682,#1433,.T.);
#3352=EDGE_CURVE('',#2681,#2683,#1434,.T.);
#3353=EDGE_CURVE('',#2681,#2684,#1435,.T.);
#3354=EDGE_CURVE('',#2685,#2683,#1436,.T.);
#3355=EDGE_CURVE('',#2684,#2685,#1437,.T.);
#3356=EDGE_CURVE('',#2680,#2679,#1438,.T.);
#3357=EDGE_CURVE('',#2682,#2678,#1439,.T.);
#3358=EDGE_CURVE('',#2686,#2685,#2233,.T.);
#3359=EDGE_CURVE('',#2686,#2687,#1440,.T.);
#3360=EDGE_CURVE('',#2687,#2684,#2234,.T.);
#3361=EDGE_CURVE('',#2688,#2689,#1441,.T.);
#3362=EDGE_CURVE('',#2688,#2690,#1442,.T.);
#3363=EDGE_CURVE('',#2691,#2690,#1443,.T.);
#3364=EDGE_CURVE('',#2689,#2691,#1444,.T.);
#3365=EDGE_CURVE('',#2689,#2670,#1445,.T.);
#3366=EDGE_CURVE('',#2671,#2691,#1446,.T.);
#3367=EDGE_CURVE('',#2688,#2692,#1447,.T.);
#3368=EDGE_CURVE('',#2693,#2692,#1448,.T.);
#3369=EDGE_CURVE('',#2690,#2693,#1449,.T.);
#3370=EDGE_CURVE('',#2692,#2694,#2235,.T.);
#3371=EDGE_CURVE('',#2694,#2695,#1450,.T.);
#3372=EDGE_CURVE('',#2693,#2695,#2236,.T.);
#3373=EDGE_CURVE('',#2696,#2697,#1451,.T.);
#3374=EDGE_CURVE('',#2696,#2698,#1452,.T.);
#3375=EDGE_CURVE('',#2699,#2698,#1453,.T.);
#3376=EDGE_CURVE('',#2697,#2699,#1454,.T.);
#3377=EDGE_CURVE('',#2697,#2700,#1455,.T.);
#3378=EDGE_CURVE('',#2701,#2699,#1456,.T.);
#3379=EDGE_CURVE('',#2700,#2701,#1457,.T.);
#3380=EDGE_CURVE('',#2696,#2702,#1458,.T.);
#3381=EDGE_CURVE('',#2703,#2702,#1459,.T.);
#3382=EDGE_CURVE('',#2698,#2703,#1460,.T.);
#3383=EDGE_CURVE('',#2704,#2701,#2237,.T.);
#3384=EDGE_CURVE('',#2704,#2705,#1461,.T.);
#3385=EDGE_CURVE('',#2705,#2700,#2238,.T.);
#3386=EDGE_CURVE('',#2702,#2706,#2239,.T.);
#3387=EDGE_CURVE('',#2706,#2707,#1462,.T.);
#3388=EDGE_CURVE('',#2703,#2707,#2240,.T.);
#3389=EDGE_CURVE('',#2708,#2709,#1463,.T.);
#3390=EDGE_CURVE('',#2708,#2710,#1464,.T.);
#3391=EDGE_CURVE('',#2711,#2710,#1465,.T.);
#3392=EDGE_CURVE('',#2709,#2711,#1466,.T.);
#3393=EDGE_CURVE('',#2709,#2694,#1467,.T.);
#3394=EDGE_CURVE('',#2695,#2711,#1468,.T.);
#3395=EDGE_CURVE('',#2708,#2705,#1469,.T.);
#3396=EDGE_CURVE('',#2710,#2704,#1470,.T.);
#3397=EDGE_CURVE('',#2712,#2713,#1471,.T.);
#3398=EDGE_CURVE('',#2712,#2714,#1472,.T.);
#3399=EDGE_CURVE('',#2715,#2714,#1473,.T.);
#3400=EDGE_CURVE('',#2713,#2715,#1474,.T.);
#3401=EDGE_CURVE('',#2713,#2706,#1475,.T.);
#3402=EDGE_CURVE('',#2707,#2715,#1476,.T.);
#3403=EDGE_CURVE('',#2712,#2637,#1477,.T.);
#3404=EDGE_CURVE('',#2714,#2636,#1478,.T.);
#3405=EDGE_CURVE('',#2716,#2717,#1479,.T.);
#3406=EDGE_CURVE('',#2716,#2718,#1480,.T.);
#3407=EDGE_CURVE('',#2719,#2718,#1481,.T.);
#3408=EDGE_CURVE('',#2717,#2719,#1482,.T.);
#3409=EDGE_CURVE('',#2717,#2654,#1483,.T.);
#3410=EDGE_CURVE('',#2655,#2719,#1484,.T.);
#3411=EDGE_CURVE('',#2716,#2687,#1485,.T.);
#3412=EDGE_CURVE('',#2718,#2686,#1486,.T.);
#3413=EDGE_CURVE('',#2720,#2721,#1487,.T.);
#3414=EDGE_CURVE('',#2722,#2720,#1488,.T.);
#3415=EDGE_CURVE('',#2723,#2722,#1489,.T.);
#3416=EDGE_CURVE('',#2721,#2723,#1490,.T.);
#3417=EDGE_CURVE('',#2724,#2725,#1491,.T.);
#3418=EDGE_CURVE('',#2726,#2725,#1492,.T.);
#3419=EDGE_CURVE('',#2727,#2726,#1493,.T.);
#3420=EDGE_CURVE('',#2724,#2727,#1494,.T.);
#3421=EDGE_CURVE('',#2728,#2723,#2241,.T.);
#3422=EDGE_CURVE('',#2728,#2729,#1495,.T.);
#3423=EDGE_CURVE('',#2729,#2721,#2242,.T.);
#3424=EDGE_CURVE('',#2725,#2730,#2243,.T.);
#3425=EDGE_CURVE('',#2730,#2731,#1496,.T.);
#3426=EDGE_CURVE('',#2726,#2731,#2244,.T.);
#3427=EDGE_CURVE('',#2732,#2727,#2245,.T.);
#3428=EDGE_CURVE('',#2732,#2733,#1497,.T.);
#3429=EDGE_CURVE('',#2733,#2724,#2246,.T.);
#3430=EDGE_CURVE('',#2720,#2734,#2247,.T.);
#3431=EDGE_CURVE('',#2734,#2735,#1498,.T.);
#3432=EDGE_CURVE('',#2722,#2735,#2248,.T.);
#3433=EDGE_CURVE('',#2733,#2730,#1499,.T.);
#3434=EDGE_CURVE('',#2731,#2732,#1500,.T.);
#3435=EDGE_CURVE('',#2736,#2737,#1501,.T.);
#3436=EDGE_CURVE('',#2738,#2737,#1502,.T.);
#3437=EDGE_CURVE('',#2739,#2738,#1503,.T.);
#3438=EDGE_CURVE('',#2736,#2739,#1504,.T.);
#3439=EDGE_CURVE('',#2737,#2740,#2249,.T.);
#3440=EDGE_CURVE('',#2740,#2741,#1505,.T.);
#3441=EDGE_CURVE('',#2738,#2741,#2250,.T.);
#3442=EDGE_CURVE('',#2742,#2739,#2251,.T.);
#3443=EDGE_CURVE('',#2742,#2743,#1506,.T.);
#3444=EDGE_CURVE('',#2743,#2736,#2252,.T.);
#3445=EDGE_CURVE('',#2743,#2740,#1507,.T.);
#3446=EDGE_CURVE('',#2741,#2742,#1508,.T.);
#3447=EDGE_CURVE('',#2744,#2745,#1509,.T.);
#3448=EDGE_CURVE('',#2746,#2745,#1510,.T.);
#3449=EDGE_CURVE('',#2747,#2746,#1511,.T.);
#3450=EDGE_CURVE('',#2744,#2747,#1512,.T.);
#3451=EDGE_CURVE('',#2745,#2748,#2253,.T.);
#3452=EDGE_CURVE('',#2748,#2749,#1513,.T.);
#3453=EDGE_CURVE('',#2746,#2749,#2254,.T.);
#3454=EDGE_CURVE('',#2750,#2747,#2255,.T.);
#3455=EDGE_CURVE('',#2750,#2751,#1514,.T.);
#3456=EDGE_CURVE('',#2751,#2744,#2256,.T.);
#3457=EDGE_CURVE('',#2751,#2748,#1515,.T.);
#3458=EDGE_CURVE('',#2749,#2750,#1516,.T.);
#3459=EDGE_CURVE('',#2752,#2753,#1517,.T.);
#3460=EDGE_CURVE('',#2754,#2753,#1518,.T.);
#3461=EDGE_CURVE('',#2755,#2754,#1519,.T.);
#3462=EDGE_CURVE('',#2752,#2755,#1520,.T.);
#3463=EDGE_CURVE('',#2753,#2756,#2257,.T.);
#3464=EDGE_CURVE('',#2756,#2757,#1521,.T.);
#3465=EDGE_CURVE('',#2754,#2757,#2258,.T.);
#3466=EDGE_CURVE('',#2758,#2755,#2259,.T.);
#3467=EDGE_CURVE('',#2758,#2759,#1522,.T.);
#3468=EDGE_CURVE('',#2759,#2752,#2260,.T.);
#3469=EDGE_CURVE('',#2759,#2756,#1523,.T.);
#3470=EDGE_CURVE('',#2757,#2758,#1524,.T.);
#3471=EDGE_CURVE('',#2760,#2761,#1525,.T.);
#3472=EDGE_CURVE('',#2762,#2761,#1526,.T.);
#3473=EDGE_CURVE('',#2763,#2762,#1527,.T.);
#3474=EDGE_CURVE('',#2760,#2763,#1528,.T.);
#3475=EDGE_CURVE('',#2761,#2764,#2261,.T.);
#3476=EDGE_CURVE('',#2764,#2765,#1529,.T.);
#3477=EDGE_CURVE('',#2762,#2765,#2262,.T.);
#3478=EDGE_CURVE('',#2766,#2763,#2263,.T.);
#3479=EDGE_CURVE('',#2766,#2767,#1530,.T.);
#3480=EDGE_CURVE('',#2767,#2760,#2264,.T.);
#3481=EDGE_CURVE('',#2767,#2764,#1531,.T.);
#3482=EDGE_CURVE('',#2765,#2766,#1532,.T.);
#3483=EDGE_CURVE('',#2734,#2729,#1533,.T.);
#3484=EDGE_CURVE('',#2735,#2728,#1534,.T.);
#3485=EDGE_CURVE('',#2768,#2768,#2265,.T.);
#3486=EDGE_CURVE('',#2768,#2769,#1535,.T.);
#3487=EDGE_CURVE('',#2769,#2769,#2266,.T.);
#4016=ORIENTED_EDGE('',*,*,#3053,.F.);
#4017=ORIENTED_EDGE('',*,*,#3054,.T.);
#4018=ORIENTED_EDGE('',*,*,#3055,.F.);
#4019=ORIENTED_EDGE('',*,*,#3056,.F.);
#4020=ORIENTED_EDGE('',*,*,#3057,.F.);
#4021=ORIENTED_EDGE('',*,*,#3056,.T.);
#4022=ORIENTED_EDGE('',*,*,#3058,.F.);
#4023=ORIENTED_EDGE('',*,*,#3059,.F.);
#4024=ORIENTED_EDGE('',*,*,#3060,.T.);
#4025=ORIENTED_EDGE('',*,*,#3061,.F.);
#4026=ORIENTED_EDGE('',*,*,#3062,.F.);
#4027=ORIENTED_EDGE('',*,*,#3054,.F.);
#4028=ORIENTED_EDGE('',*,*,#3059,.T.);
#4029=ORIENTED_EDGE('',*,*,#3063,.F.);
#4030=ORIENTED_EDGE('',*,*,#3064,.T.);
#4031=ORIENTED_EDGE('',*,*,#3065,.T.);
#4032=ORIENTED_EDGE('',*,*,#3061,.T.);
#4033=ORIENTED_EDGE('',*,*,#3066,.T.);
#4034=ORIENTED_EDGE('',*,*,#3067,.T.);
#4035=ORIENTED_EDGE('',*,*,#3068,.F.);
#4036=ORIENTED_EDGE('',*,*,#3069,.F.);
#4037=ORIENTED_EDGE('',*,*,#3070,.T.);
#4038=ORIENTED_EDGE('',*,*,#3071,.F.);
#4039=ORIENTED_EDGE('',*,*,#3072,.F.);
#4040=ORIENTED_EDGE('',*,*,#3073,.F.);
#4041=ORIENTED_EDGE('',*,*,#3072,.T.);
#4042=ORIENTED_EDGE('',*,*,#3074,.F.);
#4043=ORIENTED_EDGE('',*,*,#3075,.F.);
#4044=ORIENTED_EDGE('',*,*,#3076,.T.);
#4045=ORIENTED_EDGE('',*,*,#3064,.F.);
#4046=ORIENTED_EDGE('',*,*,#3077,.F.);
#4047=ORIENTED_EDGE('',*,*,#3070,.F.);
#4048=ORIENTED_EDGE('',*,*,#3075,.T.);
#4049=ORIENTED_EDGE('',*,*,#3078,.F.);
#4050=ORIENTED_EDGE('',*,*,#3079,.T.);
#4051=ORIENTED_EDGE('',*,*,#3080,.T.);
#4052=ORIENTED_EDGE('',*,*,#3081,.F.);
#4053=ORIENTED_EDGE('',*,*,#3082,.T.);
#4054=ORIENTED_EDGE('',*,*,#3083,.F.);
#4055=ORIENTED_EDGE('',*,*,#3084,.F.);
#4056=ORIENTED_EDGE('',*,*,#3085,.F.);
#4057=ORIENTED_EDGE('',*,*,#3084,.T.);
#4058=ORIENTED_EDGE('',*,*,#3086,.F.);
#4059=ORIENTED_EDGE('',*,*,#3087,.F.);
#4060=ORIENTED_EDGE('',*,*,#3088,.T.);
#4061=ORIENTED_EDGE('',*,*,#3079,.F.);
#4062=ORIENTED_EDGE('',*,*,#3089,.F.);
#4063=ORIENTED_EDGE('',*,*,#3082,.F.);
#4064=ORIENTED_EDGE('',*,*,#3087,.T.);
#4065=ORIENTED_EDGE('',*,*,#3090,.F.);
#4066=ORIENTED_EDGE('',*,*,#3091,.T.);
#4067=ORIENTED_EDGE('',*,*,#3092,.T.);
#4068=ORIENTED_EDGE('',*,*,#3093,.F.);
#4069=ORIENTED_EDGE('',*,*,#3094,.T.);
#4070=ORIENTED_EDGE('',*,*,#3095,.F.);
#4071=ORIENTED_EDGE('',*,*,#3096,.F.);
#4072=ORIENTED_EDGE('',*,*,#3097,.F.);
#4073=ORIENTED_EDGE('',*,*,#3096,.T.);
#4074=ORIENTED_EDGE('',*,*,#3098,.F.);
#4075=ORIENTED_EDGE('',*,*,#3099,.F.);
#4076=ORIENTED_EDGE('',*,*,#3100,.T.);
#4077=ORIENTED_EDGE('',*,*,#3091,.F.);
#4078=ORIENTED_EDGE('',*,*,#3101,.F.);
#4079=ORIENTED_EDGE('',*,*,#3094,.F.);
#4080=ORIENTED_EDGE('',*,*,#3099,.T.);
#4081=ORIENTED_EDGE('',*,*,#3102,.F.);
#4082=ORIENTED_EDGE('',*,*,#3103,.T.);
#4083=ORIENTED_EDGE('',*,*,#3104,.T.);
#4084=ORIENTED_EDGE('',*,*,#3105,.F.);
#4085=ORIENTED_EDGE('',*,*,#3106,.T.);
#4086=ORIENTED_EDGE('',*,*,#3107,.F.);
#4087=ORIENTED_EDGE('',*,*,#3108,.F.);
#4088=ORIENTED_EDGE('',*,*,#3109,.F.);
#4089=ORIENTED_EDGE('',*,*,#3108,.T.);
#4090=ORIENTED_EDGE('',*,*,#3110,.F.);
#4091=ORIENTED_EDGE('',*,*,#3111,.F.);
#4092=ORIENTED_EDGE('',*,*,#3112,.T.);
#4093=ORIENTED_EDGE('',*,*,#3103,.F.);
#4094=ORIENTED_EDGE('',*,*,#3113,.F.);
#4095=ORIENTED_EDGE('',*,*,#3106,.F.);
#4096=ORIENTED_EDGE('',*,*,#3111,.T.);
#4097=ORIENTED_EDGE('',*,*,#3114,.F.);
#4098=ORIENTED_EDGE('',*,*,#3115,.T.);
#4099=ORIENTED_EDGE('',*,*,#3116,.T.);
#4100=ORIENTED_EDGE('',*,*,#3117,.F.);
#4101=ORIENTED_EDGE('',*,*,#3118,.T.);
#4102=ORIENTED_EDGE('',*,*,#3119,.F.);
#4103=ORIENTED_EDGE('',*,*,#3120,.F.);
#4104=ORIENTED_EDGE('',*,*,#3121,.F.);
#4105=ORIENTED_EDGE('',*,*,#3120,.T.);
#4106=ORIENTED_EDGE('',*,*,#3122,.F.);
#4107=ORIENTED_EDGE('',*,*,#3123,.F.);
#4108=ORIENTED_EDGE('',*,*,#3124,.T.);
#4109=ORIENTED_EDGE('',*,*,#3125,.F.);
#4110=ORIENTED_EDGE('',*,*,#3126,.F.);
#4111=ORIENTED_EDGE('',*,*,#3118,.F.);
#4112=ORIENTED_EDGE('',*,*,#3123,.T.);
#4113=ORIENTED_EDGE('',*,*,#3127,.F.);
#4114=ORIENTED_EDGE('',*,*,#3128,.T.);
#4115=ORIENTED_EDGE('',*,*,#3129,.T.);
#4116=ORIENTED_EDGE('',*,*,#3125,.T.);
#4117=ORIENTED_EDGE('',*,*,#3130,.T.);
#4118=ORIENTED_EDGE('',*,*,#3131,.T.);
#4119=ORIENTED_EDGE('',*,*,#3132,.F.);
#4120=ORIENTED_EDGE('',*,*,#3133,.F.);
#4121=ORIENTED_EDGE('',*,*,#3134,.T.);
#4122=ORIENTED_EDGE('',*,*,#3135,.F.);
#4123=ORIENTED_EDGE('',*,*,#3136,.F.);
#4124=ORIENTED_EDGE('',*,*,#3137,.F.);
#4125=ORIENTED_EDGE('',*,*,#3136,.T.);
#4126=ORIENTED_EDGE('',*,*,#3138,.F.);
#4127=ORIENTED_EDGE('',*,*,#3131,.F.);
#4128=ORIENTED_EDGE('',*,*,#3139,.T.);
#4129=ORIENTED_EDGE('',*,*,#3115,.F.);
#4130=ORIENTED_EDGE('',*,*,#3140,.F.);
#4131=ORIENTED_EDGE('',*,*,#3134,.F.);
#4132=ORIENTED_EDGE('',*,*,#3141,.F.);
#4133=ORIENTED_EDGE('',*,*,#3142,.T.);
#4134=ORIENTED_EDGE('',*,*,#3143,.F.);
#4135=ORIENTED_EDGE('',*,*,#3144,.F.);
#4136=ORIENTED_EDGE('',*,*,#3145,.F.);
#4137=ORIENTED_EDGE('',*,*,#3144,.T.);
#4138=ORIENTED_EDGE('',*,*,#3146,.F.);
#4139=ORIENTED_EDGE('',*,*,#3147,.F.);
#4140=ORIENTED_EDGE('',*,*,#3148,.T.);
#4141=ORIENTED_EDGE('',*,*,#3128,.F.);
#4142=ORIENTED_EDGE('',*,*,#3149,.F.);
#4143=ORIENTED_EDGE('',*,*,#3142,.F.);
#4144=ORIENTED_EDGE('',*,*,#3147,.T.);
#4145=ORIENTED_EDGE('',*,*,#3150,.F.);
#4146=ORIENTED_EDGE('',*,*,#3151,.T.);
#4147=ORIENTED_EDGE('',*,*,#3152,.T.);
#4148=ORIENTED_EDGE('',*,*,#3153,.F.);
#4149=ORIENTED_EDGE('',*,*,#3154,.T.);
#4150=ORIENTED_EDGE('',*,*,#3155,.F.);
#4151=ORIENTED_EDGE('',*,*,#3156,.F.);
#4152=ORIENTED_EDGE('',*,*,#3157,.F.);
#4153=ORIENTED_EDGE('',*,*,#3156,.T.);
#4154=ORIENTED_EDGE('',*,*,#3158,.F.);
#4155=ORIENTED_EDGE('',*,*,#3159,.F.);
#4156=ORIENTED_EDGE('',*,*,#3160,.T.);
#4157=ORIENTED_EDGE('',*,*,#3161,.F.);
#4158=ORIENTED_EDGE('',*,*,#3162,.F.);
#4159=ORIENTED_EDGE('',*,*,#3154,.F.);
#4160=ORIENTED_EDGE('',*,*,#3159,.T.);
#4161=ORIENTED_EDGE('',*,*,#3163,.F.);
#4162=ORIENTED_EDGE('',*,*,#3164,.T.);
#4163=ORIENTED_EDGE('',*,*,#3165,.T.);
#4164=ORIENTED_EDGE('',*,*,#3161,.T.);
#4165=ORIENTED_EDGE('',*,*,#3166,.T.);
#4166=ORIENTED_EDGE('',*,*,#3167,.T.);
#4167=ORIENTED_EDGE('',*,*,#3168,.F.);
#4168=ORIENTED_EDGE('',*,*,#3169,.F.);
#4169=ORIENTED_EDGE('',*,*,#3170,.T.);
#4170=ORIENTED_EDGE('',*,*,#3171,.F.);
#4171=ORIENTED_EDGE('',*,*,#3172,.F.);
#4172=ORIENTED_EDGE('',*,*,#3173,.F.);
#4173=ORIENTED_EDGE('',*,*,#3172,.T.);
#4174=ORIENTED_EDGE('',*,*,#3174,.F.);
#4175=ORIENTED_EDGE('',*,*,#3175,.F.);
#4176=ORIENTED_EDGE('',*,*,#3176,.T.);
#4177=ORIENTED_EDGE('',*,*,#3177,.F.);
#4178=ORIENTED_EDGE('',*,*,#3178,.F.);
#4179=ORIENTED_EDGE('',*,*,#3170,.F.);
#4180=ORIENTED_EDGE('',*,*,#3175,.T.);
#4181=ORIENTED_EDGE('',*,*,#3179,.F.);
#4182=ORIENTED_EDGE('',*,*,#3180,.T.);
#4183=ORIENTED_EDGE('',*,*,#3181,.T.);
#4184=ORIENTED_EDGE('',*,*,#3177,.T.);
#4185=ORIENTED_EDGE('',*,*,#3182,.T.);
#4186=ORIENTED_EDGE('',*,*,#3183,.T.);
#4187=ORIENTED_EDGE('',*,*,#3184,.F.);
#4188=ORIENTED_EDGE('',*,*,#3185,.F.);
#4189=ORIENTED_EDGE('',*,*,#3186,.T.);
#4190=ORIENTED_EDGE('',*,*,#3187,.F.);
#4191=ORIENTED_EDGE('',*,*,#3188,.F.);
#4192=ORIENTED_EDGE('',*,*,#3189,.F.);
#4193=ORIENTED_EDGE('',*,*,#3188,.T.);
#4194=ORIENTED_EDGE('',*,*,#3190,.F.);
#4195=ORIENTED_EDGE('',*,*,#3183,.F.);
#4196=ORIENTED_EDGE('',*,*,#3191,.T.);
#4197=ORIENTED_EDGE('',*,*,#3164,.F.);
#4198=ORIENTED_EDGE('',*,*,#3192,.F.);
#4199=ORIENTED_EDGE('',*,*,#3186,.F.);
#4200=ORIENTED_EDGE('',*,*,#3193,.F.);
#4201=ORIENTED_EDGE('',*,*,#3194,.T.);
#4202=ORIENTED_EDGE('',*,*,#3195,.F.);
#4203=ORIENTED_EDGE('',*,*,#3196,.F.);
#4204=ORIENTED_EDGE('',*,*,#3197,.F.);
#4205=ORIENTED_EDGE('',*,*,#3196,.T.);
#4206=ORIENTED_EDGE('',*,*,#3198,.F.);
#4207=ORIENTED_EDGE('',*,*,#3167,.F.);
#4208=ORIENTED_EDGE('',*,*,#3199,.T.);
#4209=ORIENTED_EDGE('',*,*,#3151,.F.);
#4210=ORIENTED_EDGE('',*,*,#3200,.F.);
#4211=ORIENTED_EDGE('',*,*,#3194,.F.);
#4212=ORIENTED_EDGE('',*,*,#3201,.F.);
#4213=ORIENTED_EDGE('',*,*,#3202,.T.);
#4214=ORIENTED_EDGE('',*,*,#3203,.F.);
#4215=ORIENTED_EDGE('',*,*,#3204,.F.);
#4216=ORIENTED_EDGE('',*,*,#3205,.F.);
#4217=ORIENTED_EDGE('',*,*,#3204,.T.);
#4218=ORIENTED_EDGE('',*,*,#3206,.F.);
#4219=ORIENTED_EDGE('',*,*,#3207,.F.);
#4220=ORIENTED_EDGE('',*,*,#3208,.T.);
#4221=ORIENTED_EDGE('',*,*,#3180,.F.);
#4222=ORIENTED_EDGE('',*,*,#3209,.F.);
#4223=ORIENTED_EDGE('',*,*,#3202,.F.);
#4224=ORIENTED_EDGE('',*,*,#3207,.T.);
#4225=ORIENTED_EDGE('',*,*,#3210,.F.);
#4226=ORIENTED_EDGE('',*,*,#3211,.T.);
#4227=ORIENTED_EDGE('',*,*,#3212,.T.);
#4228=ORIENTED_EDGE('',*,*,#3213,.F.);
#4229=ORIENTED_EDGE('',*,*,#3214,.T.);
#4230=ORIENTED_EDGE('',*,*,#3215,.F.);
#4231=ORIENTED_EDGE('',*,*,#3216,.F.);
#4232=ORIENTED_EDGE('',*,*,#3217,.F.);
#4233=ORIENTED_EDGE('',*,*,#3216,.T.);
#4234=ORIENTED_EDGE('',*,*,#3218,.F.);
#4235=ORIENTED_EDGE('',*,*,#3219,.F.);
#4236=ORIENTED_EDGE('',*,*,#3220,.T.);
#4237=ORIENTED_EDGE('',*,*,#3211,.F.);
#4238=ORIENTED_EDGE('',*,*,#3221,.F.);
#4239=ORIENTED_EDGE('',*,*,#3214,.F.);
#4240=ORIENTED_EDGE('',*,*,#3219,.T.);
#4241=ORIENTED_EDGE('',*,*,#3222,.F.);
#4242=ORIENTED_EDGE('',*,*,#3223,.T.);
#4243=ORIENTED_EDGE('',*,*,#3224,.T.);
#4244=ORIENTED_EDGE('',*,*,#3225,.F.);
#4245=ORIENTED_EDGE('',*,*,#3226,.T.);
#4246=ORIENTED_EDGE('',*,*,#3227,.F.);
#4247=ORIENTED_EDGE('',*,*,#3228,.F.);
#4248=ORIENTED_EDGE('',*,*,#3229,.F.);
#4249=ORIENTED_EDGE('',*,*,#3228,.T.);
#4250=ORIENTED_EDGE('',*,*,#3230,.F.);
#4251=ORIENTED_EDGE('',*,*,#3231,.F.);
#4252=ORIENTED_EDGE('',*,*,#3232,.T.);
#4253=ORIENTED_EDGE('',*,*,#3233,.F.);
#4254=ORIENTED_EDGE('',*,*,#3234,.F.);
#4255=ORIENTED_EDGE('',*,*,#3226,.F.);
#4256=ORIENTED_EDGE('',*,*,#3231,.T.);
#4257=ORIENTED_EDGE('',*,*,#3235,.F.);
#4258=ORIENTED_EDGE('',*,*,#3236,.T.);
#4259=ORIENTED_EDGE('',*,*,#3237,.T.);
#4260=ORIENTED_EDGE('',*,*,#3233,.T.);
#4261=ORIENTED_EDGE('',*,*,#3238,.T.);
#4262=ORIENTED_EDGE('',*,*,#3239,.T.);
#4263=ORIENTED_EDGE('',*,*,#3240,.F.);
#4264=ORIENTED_EDGE('',*,*,#3241,.F.);
#4265=ORIENTED_EDGE('',*,*,#3242,.T.);
#4266=ORIENTED_EDGE('',*,*,#3243,.F.);
#4267=ORIENTED_EDGE('',*,*,#3244,.F.);
#4268=ORIENTED_EDGE('',*,*,#3245,.F.);
#4269=ORIENTED_EDGE('',*,*,#3244,.T.);
#4270=ORIENTED_EDGE('',*,*,#3246,.F.);
#4271=ORIENTED_EDGE('',*,*,#3247,.F.);
#4272=ORIENTED_EDGE('',*,*,#3248,.T.);
#4273=ORIENTED_EDGE('',*,*,#3223,.F.);
#4274=ORIENTED_EDGE('',*,*,#3249,.F.);
#4275=ORIENTED_EDGE('',*,*,#3242,.F.);
#4276=ORIENTED_EDGE('',*,*,#3247,.T.);
#4277=ORIENTED_EDGE('',*,*,#3250,.F.);
#4278=ORIENTED_EDGE('',*,*,#3251,.T.);
#4279=ORIENTED_EDGE('',*,*,#3252,.T.);
#4280=ORIENTED_EDGE('',*,*,#3253,.F.);
#4281=ORIENTED_EDGE('',*,*,#3254,.T.);
#4282=ORIENTED_EDGE('',*,*,#3255,.F.);
#4283=ORIENTED_EDGE('',*,*,#3256,.F.);
#4284=ORIENTED_EDGE('',*,*,#3257,.F.);
#4285=ORIENTED_EDGE('',*,*,#3256,.T.);
#4286=ORIENTED_EDGE('',*,*,#3258,.F.);
#4287=ORIENTED_EDGE('',*,*,#3259,.F.);
#4288=ORIENTED_EDGE('',*,*,#3260,.T.);
#4289=ORIENTED_EDGE('',*,*,#3251,.F.);
#4290=ORIENTED_EDGE('',*,*,#3261,.F.);
#4291=ORIENTED_EDGE('',*,*,#3254,.F.);
#4292=ORIENTED_EDGE('',*,*,#3259,.T.);
#4293=ORIENTED_EDGE('',*,*,#3262,.F.);
#4294=ORIENTED_EDGE('',*,*,#3263,.T.);
#4295=ORIENTED_EDGE('',*,*,#3264,.T.);
#4296=ORIENTED_EDGE('',*,*,#3265,.F.);
#4297=ORIENTED_EDGE('',*,*,#3266,.T.);
#4298=ORIENTED_EDGE('',*,*,#3267,.F.);
#4299=ORIENTED_EDGE('',*,*,#3268,.F.);
#4300=ORIENTED_EDGE('',*,*,#3269,.F.);
#4301=ORIENTED_EDGE('',*,*,#3268,.T.);
#4302=ORIENTED_EDGE('',*,*,#3270,.F.);
#4303=ORIENTED_EDGE('',*,*,#3239,.F.);
#4304=ORIENTED_EDGE('',*,*,#3271,.T.);
#4305=ORIENTED_EDGE('',*,*,#3263,.F.);
#4306=ORIENTED_EDGE('',*,*,#3272,.F.);
#4307=ORIENTED_EDGE('',*,*,#3266,.F.);
#4308=ORIENTED_EDGE('',*,*,#3273,.F.);
#4309=ORIENTED_EDGE('',*,*,#3274,.T.);
#4310=ORIENTED_EDGE('',*,*,#3275,.F.);
#4311=ORIENTED_EDGE('',*,*,#3276,.F.);
#4312=ORIENTED_EDGE('',*,*,#3277,.F.);
#4313=ORIENTED_EDGE('',*,*,#3276,.T.);
#4314=ORIENTED_EDGE('',*,*,#3278,.F.);
#4315=ORIENTED_EDGE('',*,*,#3279,.F.);
#4316=ORIENTED_EDGE('',*,*,#3280,.T.);
#4317=ORIENTED_EDGE('',*,*,#3281,.F.);
#4318=ORIENTED_EDGE('',*,*,#3282,.F.);
#4319=ORIENTED_EDGE('',*,*,#3274,.F.);
#4320=ORIENTED_EDGE('',*,*,#3279,.T.);
#4321=ORIENTED_EDGE('',*,*,#3283,.F.);
#4322=ORIENTED_EDGE('',*,*,#3284,.T.);
#4323=ORIENTED_EDGE('',*,*,#3285,.T.);
#4324=ORIENTED_EDGE('',*,*,#3281,.T.);
#4325=ORIENTED_EDGE('',*,*,#3286,.T.);
#4326=ORIENTED_EDGE('',*,*,#3287,.T.);
#4327=ORIENTED_EDGE('',*,*,#3288,.F.);
#4328=ORIENTED_EDGE('',*,*,#3289,.F.);
#4329=ORIENTED_EDGE('',*,*,#3290,.T.);
#4330=ORIENTED_EDGE('',*,*,#3291,.F.);
#4331=ORIENTED_EDGE('',*,*,#3292,.F.);
#4332=ORIENTED_EDGE('',*,*,#3293,.F.);
#4333=ORIENTED_EDGE('',*,*,#3292,.T.);
#4334=ORIENTED_EDGE('',*,*,#3294,.F.);
#4335=ORIENTED_EDGE('',*,*,#3287,.F.);
#4336=ORIENTED_EDGE('',*,*,#3295,.T.);
#4337=ORIENTED_EDGE('',*,*,#3236,.F.);
#4338=ORIENTED_EDGE('',*,*,#3296,.F.);
#4339=ORIENTED_EDGE('',*,*,#3290,.F.);
#4340=ORIENTED_EDGE('',*,*,#3297,.F.);
#4341=ORIENTED_EDGE('',*,*,#3298,.T.);
#4342=ORIENTED_EDGE('',*,*,#3299,.F.);
#4343=ORIENTED_EDGE('',*,*,#3300,.F.);
#4344=ORIENTED_EDGE('',*,*,#3301,.F.);
#4345=ORIENTED_EDGE('',*,*,#3300,.T.);
#4346=ORIENTED_EDGE('',*,*,#3302,.F.);
#4347=ORIENTED_EDGE('',*,*,#3303,.F.);
#4348=ORIENTED_EDGE('',*,*,#3304,.T.);
#4349=ORIENTED_EDGE('',*,*,#3305,.F.);
#4350=ORIENTED_EDGE('',*,*,#3306,.F.);
#4351=ORIENTED_EDGE('',*,*,#3298,.F.);
#4352=ORIENTED_EDGE('',*,*,#3303,.T.);
#4353=ORIENTED_EDGE('',*,*,#3307,.F.);
#4354=ORIENTED_EDGE('',*,*,#3308,.T.);
#4355=ORIENTED_EDGE('',*,*,#3309,.T.);
#4356=ORIENTED_EDGE('',*,*,#3305,.T.);
#4357=ORIENTED_EDGE('',*,*,#3310,.T.);
#4358=ORIENTED_EDGE('',*,*,#3311,.T.);
#4359=ORIENTED_EDGE('',*,*,#3312,.F.);
#4360=ORIENTED_EDGE('',*,*,#3313,.F.);
#4361=ORIENTED_EDGE('',*,*,#3314,.T.);
#4362=ORIENTED_EDGE('',*,*,#3315,.F.);
#4363=ORIENTED_EDGE('',*,*,#3316,.F.);
#4364=ORIENTED_EDGE('',*,*,#3317,.F.);
#4365=ORIENTED_EDGE('',*,*,#3316,.T.);
#4366=ORIENTED_EDGE('',*,*,#3318,.F.);
#4367=ORIENTED_EDGE('',*,*,#3067,.F.);
#4368=ORIENTED_EDGE('',*,*,#3319,.T.);
#4369=ORIENTED_EDGE('',*,*,#3308,.F.);
#4370=ORIENTED_EDGE('',*,*,#3320,.F.);
#4371=ORIENTED_EDGE('',*,*,#3314,.F.);
#4372=ORIENTED_EDGE('',*,*,#3321,.F.);
#4373=ORIENTED_EDGE('',*,*,#3322,.T.);
#4374=ORIENTED_EDGE('',*,*,#3323,.F.);
#4375=ORIENTED_EDGE('',*,*,#3324,.F.);
#4376=ORIENTED_EDGE('',*,*,#3325,.F.);
#4377=ORIENTED_EDGE('',*,*,#3324,.T.);
#4378=ORIENTED_EDGE('',*,*,#3326,.F.);
#4379=ORIENTED_EDGE('',*,*,#3327,.F.);
#4380=ORIENTED_EDGE('',*,*,#3328,.T.);
#4381=ORIENTED_EDGE('',*,*,#3329,.F.);
#4382=ORIENTED_EDGE('',*,*,#3330,.F.);
#4383=ORIENTED_EDGE('',*,*,#3322,.F.);
#4384=ORIENTED_EDGE('',*,*,#3327,.T.);
#4385=ORIENTED_EDGE('',*,*,#3331,.F.);
#4386=ORIENTED_EDGE('',*,*,#3332,.T.);
#4387=ORIENTED_EDGE('',*,*,#3333,.T.);
#4388=ORIENTED_EDGE('',*,*,#3329,.T.);
#4389=ORIENTED_EDGE('',*,*,#3334,.T.);
#4390=ORIENTED_EDGE('',*,*,#3335,.T.);
#4391=ORIENTED_EDGE('',*,*,#3336,.F.);
#4392=ORIENTED_EDGE('',*,*,#3337,.F.);
#4393=ORIENTED_EDGE('',*,*,#3338,.T.);
#4394=ORIENTED_EDGE('',*,*,#3339,.F.);
#4395=ORIENTED_EDGE('',*,*,#3340,.F.);
#4396=ORIENTED_EDGE('',*,*,#3341,.F.);
#4397=ORIENTED_EDGE('',*,*,#3340,.T.);
#4398=ORIENTED_EDGE('',*,*,#3342,.F.);
#4399=ORIENTED_EDGE('',*,*,#3343,.F.);
#4400=ORIENTED_EDGE('',*,*,#3344,.T.);
#4401=ORIENTED_EDGE('',*,*,#3332,.F.);
#4402=ORIENTED_EDGE('',*,*,#3345,.F.);
#4403=ORIENTED_EDGE('',*,*,#3338,.F.);
#4404=ORIENTED_EDGE('',*,*,#3343,.T.);
#4405=ORIENTED_EDGE('',*,*,#3346,.F.);
#4406=ORIENTED_EDGE('',*,*,#3347,.T.);
#4407=ORIENTED_EDGE('',*,*,#3348,.T.);
#4408=ORIENTED_EDGE('',*,*,#3349,.F.);
#4409=ORIENTED_EDGE('',*,*,#3350,.T.);
#4410=ORIENTED_EDGE('',*,*,#3351,.F.);
#4411=ORIENTED_EDGE('',*,*,#3352,.F.);
#4412=ORIENTED_EDGE('',*,*,#3353,.F.);
#4413=ORIENTED_EDGE('',*,*,#3352,.T.);
#4414=ORIENTED_EDGE('',*,*,#3354,.F.);
#4415=ORIENTED_EDGE('',*,*,#3355,.F.);
#4416=ORIENTED_EDGE('',*,*,#3356,.T.);
#4417=ORIENTED_EDGE('',*,*,#3347,.F.);
#4418=ORIENTED_EDGE('',*,*,#3357,.F.);
#4419=ORIENTED_EDGE('',*,*,#3350,.F.);
#4420=ORIENTED_EDGE('',*,*,#3355,.T.);
#4421=ORIENTED_EDGE('',*,*,#3358,.F.);
#4422=ORIENTED_EDGE('',*,*,#3359,.T.);
#4423=ORIENTED_EDGE('',*,*,#3360,.T.);
#4424=ORIENTED_EDGE('',*,*,#3361,.F.);
#4425=ORIENTED_EDGE('',*,*,#3362,.T.);
#4426=ORIENTED_EDGE('',*,*,#3363,.F.);
#4427=ORIENTED_EDGE('',*,*,#3364,.F.);
#4428=ORIENTED_EDGE('',*,*,#3365,.F.);
#4429=ORIENTED_EDGE('',*,*,#3364,.T.);
#4430=ORIENTED_EDGE('',*,*,#3366,.F.);
#4431=ORIENTED_EDGE('',*,*,#3335,.F.);
#4432=ORIENTED_EDGE('',*,*,#3367,.T.);
#4433=ORIENTED_EDGE('',*,*,#3368,.F.);
#4434=ORIENTED_EDGE('',*,*,#3369,.F.);
#4435=ORIENTED_EDGE('',*,*,#3362,.F.);
#4436=ORIENTED_EDGE('',*,*,#3368,.T.);
#4437=ORIENTED_EDGE('',*,*,#3370,.T.);
#4438=ORIENTED_EDGE('',*,*,#3371,.T.);
#4439=ORIENTED_EDGE('',*,*,#3372,.F.);
#4440=ORIENTED_EDGE('',*,*,#3373,.F.);
#4441=ORIENTED_EDGE('',*,*,#3374,.T.);
#4442=ORIENTED_EDGE('',*,*,#3375,.F.);
#4443=ORIENTED_EDGE('',*,*,#3376,.F.);
#4444=ORIENTED_EDGE('',*,*,#3377,.F.);
#4445=ORIENTED_EDGE('',*,*,#3376,.T.);
#4446=ORIENTED_EDGE('',*,*,#3378,.F.);
#4447=ORIENTED_EDGE('',*,*,#3379,.F.);
#4448=ORIENTED_EDGE('',*,*,#3380,.T.);
#4449=ORIENTED_EDGE('',*,*,#3381,.F.);
#4450=ORIENTED_EDGE('',*,*,#3382,.F.);
#4451=ORIENTED_EDGE('',*,*,#3374,.F.);
#4452=ORIENTED_EDGE('',*,*,#3379,.T.);
#4453=ORIENTED_EDGE('',*,*,#3383,.F.);
#4454=ORIENTED_EDGE('',*,*,#3384,.T.);
#4455=ORIENTED_EDGE('',*,*,#3385,.T.);
#4456=ORIENTED_EDGE('',*,*,#3381,.T.);
#4457=ORIENTED_EDGE('',*,*,#3386,.T.);
#4458=ORIENTED_EDGE('',*,*,#3387,.T.);
#4459=ORIENTED_EDGE('',*,*,#3388,.F.);
#4460=ORIENTED_EDGE('',*,*,#3389,.F.);
#4461=ORIENTED_EDGE('',*,*,#3390,.T.);
#4462=ORIENTED_EDGE('',*,*,#3391,.F.);
#4463=ORIENTED_EDGE('',*,*,#3392,.F.);
#4464=ORIENTED_EDGE('',*,*,#3393,.F.);
#4465=ORIENTED_EDGE('',*,*,#3392,.T.);
#4466=ORIENTED_EDGE('',*,*,#3394,.F.);
#4467=ORIENTED_EDGE('',*,*,#3371,.F.);
#4468=ORIENTED_EDGE('',*,*,#3395,.T.);
#4469=ORIENTED_EDGE('',*,*,#3384,.F.);
#4470=ORIENTED_EDGE('',*,*,#3396,.F.);
#4471=ORIENTED_EDGE('',*,*,#3390,.F.);
#4472=ORIENTED_EDGE('',*,*,#3397,.F.);
#4473=ORIENTED_EDGE('',*,*,#3398,.T.);
#4474=ORIENTED_EDGE('',*,*,#3399,.F.);
#4475=ORIENTED_EDGE('',*,*,#3400,.F.);
#4476=ORIENTED_EDGE('',*,*,#3401,.F.);
#4477=ORIENTED_EDGE('',*,*,#3400,.T.);
#4478=ORIENTED_EDGE('',*,*,#3402,.F.);
#4479=ORIENTED_EDGE('',*,*,#3387,.F.);
#4480=ORIENTED_EDGE('',*,*,#3403,.T.);
#4481=ORIENTED_EDGE('',*,*,#3284,.F.);
#4482=ORIENTED_EDGE('',*,*,#3404,.F.);
#4483=ORIENTED_EDGE('',*,*,#3398,.F.);
#4484=ORIENTED_EDGE('',*,*,#3405,.F.);
#4485=ORIENTED_EDGE('',*,*,#3406,.T.);
#4486=ORIENTED_EDGE('',*,*,#3407,.F.);
#4487=ORIENTED_EDGE('',*,*,#3408,.F.);
#4488=ORIENTED_EDGE('',*,*,#3409,.F.);
#4489=ORIENTED_EDGE('',*,*,#3408,.T.);
#4490=ORIENTED_EDGE('',*,*,#3410,.F.);
#4491=ORIENTED_EDGE('',*,*,#3311,.F.);
#4492=ORIENTED_EDGE('',*,*,#3411,.T.);
#4493=ORIENTED_EDGE('',*,*,#3359,.F.);
#4494=ORIENTED_EDGE('',*,*,#3412,.F.);
#4495=ORIENTED_EDGE('',*,*,#3406,.F.);
#4496=ORIENTED_EDGE('',*,*,#3413,.F.);
#4497=ORIENTED_EDGE('',*,*,#3414,.F.);
#4498=ORIENTED_EDGE('',*,*,#3415,.F.);
#4499=ORIENTED_EDGE('',*,*,#3416,.F.);
#4500=ORIENTED_EDGE('',*,*,#3417,.T.);
#4501=ORIENTED_EDGE('',*,*,#3418,.F.);
#4502=ORIENTED_EDGE('',*,*,#3419,.F.);
#4503=ORIENTED_EDGE('',*,*,#3420,.F.);
#4504=ORIENTED_EDGE('',*,*,#3416,.T.);
#4505=ORIENTED_EDGE('',*,*,#3421,.F.);
#4506=ORIENTED_EDGE('',*,*,#3422,.T.);
#4507=ORIENTED_EDGE('',*,*,#3423,.T.);
#4508=ORIENTED_EDGE('',*,*,#3418,.T.);
#4509=ORIENTED_EDGE('',*,*,#3424,.T.);
#4510=ORIENTED_EDGE('',*,*,#3425,.T.);
#4511=ORIENTED_EDGE('',*,*,#3426,.F.);
#4512=ORIENTED_EDGE('',*,*,#3420,.T.);
#4513=ORIENTED_EDGE('',*,*,#3427,.F.);
#4514=ORIENTED_EDGE('',*,*,#3428,.T.);
#4515=ORIENTED_EDGE('',*,*,#3429,.T.);
#4516=ORIENTED_EDGE('',*,*,#3414,.T.);
#4517=ORIENTED_EDGE('',*,*,#3430,.T.);
#4518=ORIENTED_EDGE('',*,*,#3431,.T.);
#4519=ORIENTED_EDGE('',*,*,#3432,.F.);
#4520=ORIENTED_EDGE('',*,*,#3433,.F.);
#4521=ORIENTED_EDGE('',*,*,#3428,.F.);
#4522=ORIENTED_EDGE('',*,*,#3434,.F.);
#4523=ORIENTED_EDGE('',*,*,#3425,.F.);
#4524=ORIENTED_EDGE('',*,*,#3435,.T.);
#4525=ORIENTED_EDGE('',*,*,#3436,.F.);
#4526=ORIENTED_EDGE('',*,*,#3437,.F.);
#4527=ORIENTED_EDGE('',*,*,#3438,.F.);
#4528=ORIENTED_EDGE('',*,*,#3436,.T.);
#4529=ORIENTED_EDGE('',*,*,#3439,.T.);
#4530=ORIENTED_EDGE('',*,*,#3440,.T.);
#4531=ORIENTED_EDGE('',*,*,#3441,.F.);
#4532=ORIENTED_EDGE('',*,*,#3438,.T.);
#4533=ORIENTED_EDGE('',*,*,#3442,.F.);
#4534=ORIENTED_EDGE('',*,*,#3443,.T.);
#4535=ORIENTED_EDGE('',*,*,#3444,.T.);
#4536=ORIENTED_EDGE('',*,*,#3445,.F.);
#4537=ORIENTED_EDGE('',*,*,#3443,.F.);
#4538=ORIENTED_EDGE('',*,*,#3446,.F.);
#4539=ORIENTED_EDGE('',*,*,#3440,.F.);
#4540=ORIENTED_EDGE('',*,*,#3447,.T.);
#4541=ORIENTED_EDGE('',*,*,#3448,.F.);
#4542=ORIENTED_EDGE('',*,*,#3449,.F.);
#4543=ORIENTED_EDGE('',*,*,#3450,.F.);
#4544=ORIENTED_EDGE('',*,*,#3448,.T.);
#4545=ORIENTED_EDGE('',*,*,#3451,.T.);
#4546=ORIENTED_EDGE('',*,*,#3452,.T.);
#4547=ORIENTED_EDGE('',*,*,#3453,.F.);
#4548=ORIENTED_EDGE('',*,*,#3450,.T.);
#4549=ORIENTED_EDGE('',*,*,#3454,.F.);
#4550=ORIENTED_EDGE('',*,*,#3455,.T.);
#4551=ORIENTED_EDGE('',*,*,#3456,.T.);
#4552=ORIENTED_EDGE('',*,*,#3457,.F.);
#4553=ORIENTED_EDGE('',*,*,#3455,.F.);
#4554=ORIENTED_EDGE('',*,*,#3458,.F.);
#4555=ORIENTED_EDGE('',*,*,#3452,.F.);
#4556=ORIENTED_EDGE('',*,*,#3459,.T.);
#4557=ORIENTED_EDGE('',*,*,#3460,.F.);
#4558=ORIENTED_EDGE('',*,*,#3461,.F.);
#4559=ORIENTED_EDGE('',*,*,#3462,.F.);
#4560=ORIENTED_EDGE('',*,*,#3460,.T.);
#4561=ORIENTED_EDGE('',*,*,#3463,.T.);
#4562=ORIENTED_EDGE('',*,*,#3464,.T.);
#4563=ORIENTED_EDGE('',*,*,#3465,.F.);
#4564=ORIENTED_EDGE('',*,*,#3462,.T.);
#4565=ORIENTED_EDGE('',*,*,#3466,.F.);
#4566=ORIENTED_EDGE('',*,*,#3467,.T.);
#4567=ORIENTED_EDGE('',*,*,#3468,.T.);
#4568=ORIENTED_EDGE('',*,*,#3469,.F.);
#4569=ORIENTED_EDGE('',*,*,#3467,.F.);
#4570=ORIENTED_EDGE('',*,*,#3470,.F.);
#4571=ORIENTED_EDGE('',*,*,#3464,.F.);
#4572=ORIENTED_EDGE('',*,*,#3471,.T.);
#4573=ORIENTED_EDGE('',*,*,#3472,.F.);
#4574=ORIENTED_EDGE('',*,*,#3473,.F.);
#4575=ORIENTED_EDGE('',*,*,#3474,.F.);
#4576=ORIENTED_EDGE('',*,*,#3472,.T.);
#4577=ORIENTED_EDGE('',*,*,#3475,.T.);
#4578=ORIENTED_EDGE('',*,*,#3476,.T.);
#4579=ORIENTED_EDGE('',*,*,#3477,.F.);
#4580=ORIENTED_EDGE('',*,*,#3474,.T.);
#4581=ORIENTED_EDGE('',*,*,#3478,.F.);
#4582=ORIENTED_EDGE('',*,*,#3479,.T.);
#4583=ORIENTED_EDGE('',*,*,#3480,.T.);
#4584=ORIENTED_EDGE('',*,*,#3481,.F.);
#4585=ORIENTED_EDGE('',*,*,#3479,.F.);
#4586=ORIENTED_EDGE('',*,*,#3482,.F.);
#4587=ORIENTED_EDGE('',*,*,#3476,.F.);
#4588=ORIENTED_EDGE('',*,*,#3483,.T.);
#4589=ORIENTED_EDGE('',*,*,#3422,.F.);
#4590=ORIENTED_EDGE('',*,*,#3484,.F.);
#4591=ORIENTED_EDGE('',*,*,#3431,.F.);
#4592=ORIENTED_EDGE('',*,*,#3485,.T.);
#4593=ORIENTED_EDGE('',*,*,#3486,.T.);
#4594=ORIENTED_EDGE('',*,*,#3487,.F.);
#4595=ORIENTED_EDGE('',*,*,#3486,.F.);
#4596=ORIENTED_EDGE('',*,*,#3358,.T.);
#4597=ORIENTED_EDGE('',*,*,#3354,.T.);
#4598=ORIENTED_EDGE('',*,*,#3351,.T.);
#4599=ORIENTED_EDGE('',*,*,#3357,.T.);
#4600=ORIENTED_EDGE('',*,*,#3346,.T.);
#4601=ORIENTED_EDGE('',*,*,#3342,.T.);
#4602=ORIENTED_EDGE('',*,*,#3339,.T.);
#4603=ORIENTED_EDGE('',*,*,#3345,.T.);
#4604=ORIENTED_EDGE('',*,*,#3331,.T.);
#4605=ORIENTED_EDGE('',*,*,#3326,.T.);
#4606=ORIENTED_EDGE('',*,*,#3323,.T.);
#4607=ORIENTED_EDGE('',*,*,#3330,.T.);
#4608=ORIENTED_EDGE('',*,*,#3336,.T.);
#4609=ORIENTED_EDGE('',*,*,#3366,.T.);
#4610=ORIENTED_EDGE('',*,*,#3363,.T.);
#4611=ORIENTED_EDGE('',*,*,#3369,.T.);
#4612=ORIENTED_EDGE('',*,*,#3372,.T.);
#4613=ORIENTED_EDGE('',*,*,#3394,.T.);
#4614=ORIENTED_EDGE('',*,*,#3391,.T.);
#4615=ORIENTED_EDGE('',*,*,#3396,.T.);
#4616=ORIENTED_EDGE('',*,*,#3383,.T.);
#4617=ORIENTED_EDGE('',*,*,#3378,.T.);
#4618=ORIENTED_EDGE('',*,*,#3375,.T.);
#4619=ORIENTED_EDGE('',*,*,#3382,.T.);
#4620=ORIENTED_EDGE('',*,*,#3388,.T.);
#4621=ORIENTED_EDGE('',*,*,#3402,.T.);
#4622=ORIENTED_EDGE('',*,*,#3399,.T.);
#4623=ORIENTED_EDGE('',*,*,#3404,.T.);
#4624=ORIENTED_EDGE('',*,*,#3283,.T.);
#4625=ORIENTED_EDGE('',*,*,#3278,.T.);
#4626=ORIENTED_EDGE('',*,*,#3275,.T.);
#4627=ORIENTED_EDGE('',*,*,#3282,.T.);
#4628=ORIENTED_EDGE('',*,*,#3288,.T.);
#4629=ORIENTED_EDGE('',*,*,#3294,.T.);
#4630=ORIENTED_EDGE('',*,*,#3291,.T.);
#4631=ORIENTED_EDGE('',*,*,#3296,.T.);
#4632=ORIENTED_EDGE('',*,*,#3235,.T.);
#4633=ORIENTED_EDGE('',*,*,#3230,.T.);
#4634=ORIENTED_EDGE('',*,*,#3227,.T.);
#4635=ORIENTED_EDGE('',*,*,#3234,.T.);
#4636=ORIENTED_EDGE('',*,*,#3240,.T.);
#4637=ORIENTED_EDGE('',*,*,#3270,.T.);
#4638=ORIENTED_EDGE('',*,*,#3267,.T.);
#4639=ORIENTED_EDGE('',*,*,#3272,.T.);
#4640=ORIENTED_EDGE('',*,*,#3262,.T.);
#4641=ORIENTED_EDGE('',*,*,#3258,.T.);
#4642=ORIENTED_EDGE('',*,*,#3255,.T.);
#4643=ORIENTED_EDGE('',*,*,#3261,.T.);
#4644=ORIENTED_EDGE('',*,*,#3250,.T.);
#4645=ORIENTED_EDGE('',*,*,#3246,.T.);
#4646=ORIENTED_EDGE('',*,*,#3243,.T.);
#4647=ORIENTED_EDGE('',*,*,#3249,.T.);
#4648=ORIENTED_EDGE('',*,*,#3222,.T.);
#4649=ORIENTED_EDGE('',*,*,#3218,.T.);
#4650=ORIENTED_EDGE('',*,*,#3215,.T.);
#4651=ORIENTED_EDGE('',*,*,#3221,.T.);
#4652=ORIENTED_EDGE('',*,*,#3210,.T.);
#4653=ORIENTED_EDGE('',*,*,#3206,.T.);
#4654=ORIENTED_EDGE('',*,*,#3203,.T.);
#4655=ORIENTED_EDGE('',*,*,#3209,.T.);
#4656=ORIENTED_EDGE('',*,*,#3179,.T.);
#4657=ORIENTED_EDGE('',*,*,#3174,.T.);
#4658=ORIENTED_EDGE('',*,*,#3171,.T.);
#4659=ORIENTED_EDGE('',*,*,#3178,.T.);
#4660=ORIENTED_EDGE('',*,*,#3184,.T.);
#4661=ORIENTED_EDGE('',*,*,#3190,.T.);
#4662=ORIENTED_EDGE('',*,*,#3187,.T.);
#4663=ORIENTED_EDGE('',*,*,#3192,.T.);
#4664=ORIENTED_EDGE('',*,*,#3163,.T.);
#4665=ORIENTED_EDGE('',*,*,#3158,.T.);
#4666=ORIENTED_EDGE('',*,*,#3155,.T.);
#4667=ORIENTED_EDGE('',*,*,#3162,.T.);
#4668=ORIENTED_EDGE('',*,*,#3168,.T.);
#4669=ORIENTED_EDGE('',*,*,#3198,.T.);
#4670=ORIENTED_EDGE('',*,*,#3195,.T.);
#4671=ORIENTED_EDGE('',*,*,#3200,.T.);
#4672=ORIENTED_EDGE('',*,*,#3150,.T.);
#4673=ORIENTED_EDGE('',*,*,#3146,.T.);
#4674=ORIENTED_EDGE('',*,*,#3143,.T.);
#4675=ORIENTED_EDGE('',*,*,#3149,.T.);
#4676=ORIENTED_EDGE('',*,*,#3127,.T.);
#4677=ORIENTED_EDGE('',*,*,#3122,.T.);
#4678=ORIENTED_EDGE('',*,*,#3119,.T.);
#4679=ORIENTED_EDGE('',*,*,#3126,.T.);
#4680=ORIENTED_EDGE('',*,*,#3132,.T.);
#4681=ORIENTED_EDGE('',*,*,#3138,.T.);
#4682=ORIENTED_EDGE('',*,*,#3135,.T.);
#4683=ORIENTED_EDGE('',*,*,#3140,.T.);
#4684=ORIENTED_EDGE('',*,*,#3114,.T.);
#4685=ORIENTED_EDGE('',*,*,#3110,.T.);
#4686=ORIENTED_EDGE('',*,*,#3107,.T.);
#4687=ORIENTED_EDGE('',*,*,#3113,.T.);
#4688=ORIENTED_EDGE('',*,*,#3102,.T.);
#4689=ORIENTED_EDGE('',*,*,#3098,.T.);
#4690=ORIENTED_EDGE('',*,*,#3095,.T.);
#4691=ORIENTED_EDGE('',*,*,#3101,.T.);
#4692=ORIENTED_EDGE('',*,*,#3090,.T.);
#4693=ORIENTED_EDGE('',*,*,#3086,.T.);
#4694=ORIENTED_EDGE('',*,*,#3083,.T.);
#4695=ORIENTED_EDGE('',*,*,#3089,.T.);
#4696=ORIENTED_EDGE('',*,*,#3078,.T.);
#4697=ORIENTED_EDGE('',*,*,#3074,.T.);
#4698=ORIENTED_EDGE('',*,*,#3071,.T.);
#4699=ORIENTED_EDGE('',*,*,#3077,.T.);
#4700=ORIENTED_EDGE('',*,*,#3063,.T.);
#4701=ORIENTED_EDGE('',*,*,#3058,.T.);
#4702=ORIENTED_EDGE('',*,*,#3055,.T.);
#4703=ORIENTED_EDGE('',*,*,#3062,.T.);
#4704=ORIENTED_EDGE('',*,*,#3068,.T.);
#4705=ORIENTED_EDGE('',*,*,#3318,.T.);
#4706=ORIENTED_EDGE('',*,*,#3315,.T.);
#4707=ORIENTED_EDGE('',*,*,#3320,.T.);
#4708=ORIENTED_EDGE('',*,*,#3307,.T.);
#4709=ORIENTED_EDGE('',*,*,#3302,.T.);
#4710=ORIENTED_EDGE('',*,*,#3299,.T.);
#4711=ORIENTED_EDGE('',*,*,#3306,.T.);
#4712=ORIENTED_EDGE('',*,*,#3312,.T.);
#4713=ORIENTED_EDGE('',*,*,#3410,.T.);
#4714=ORIENTED_EDGE('',*,*,#3407,.T.);
#4715=ORIENTED_EDGE('',*,*,#3412,.T.);
#4716=ORIENTED_EDGE('',*,*,#3426,.T.);
#4717=ORIENTED_EDGE('',*,*,#3434,.T.);
#4718=ORIENTED_EDGE('',*,*,#3427,.T.);
#4719=ORIENTED_EDGE('',*,*,#3419,.T.);
#4720=ORIENTED_EDGE('',*,*,#3441,.T.);
#4721=ORIENTED_EDGE('',*,*,#3446,.T.);
#4722=ORIENTED_EDGE('',*,*,#3442,.T.);
#4723=ORIENTED_EDGE('',*,*,#3437,.T.);
#4724=ORIENTED_EDGE('',*,*,#3453,.T.);
#4725=ORIENTED_EDGE('',*,*,#3458,.T.);
#4726=ORIENTED_EDGE('',*,*,#3454,.T.);
#4727=ORIENTED_EDGE('',*,*,#3449,.T.);
#4728=ORIENTED_EDGE('',*,*,#3465,.T.);
#4729=ORIENTED_EDGE('',*,*,#3470,.T.);
#4730=ORIENTED_EDGE('',*,*,#3466,.T.);
#4731=ORIENTED_EDGE('',*,*,#3461,.T.);
#4732=ORIENTED_EDGE('',*,*,#3477,.T.);
#4733=ORIENTED_EDGE('',*,*,#3482,.T.);
#4734=ORIENTED_EDGE('',*,*,#3478,.T.);
#4735=ORIENTED_EDGE('',*,*,#3473,.T.);
#4736=ORIENTED_EDGE('',*,*,#3487,.T.);
#4737=ORIENTED_EDGE('',*,*,#3415,.T.);
#4738=ORIENTED_EDGE('',*,*,#3432,.T.);
#4739=ORIENTED_EDGE('',*,*,#3484,.T.);
#4740=ORIENTED_EDGE('',*,*,#3421,.T.);
#4741=ORIENTED_EDGE('',*,*,#3360,.F.);
#4742=ORIENTED_EDGE('',*,*,#3411,.F.);
#4743=ORIENTED_EDGE('',*,*,#3405,.T.);
#4744=ORIENTED_EDGE('',*,*,#3409,.T.);
#4745=ORIENTED_EDGE('',*,*,#3310,.F.);
#4746=ORIENTED_EDGE('',*,*,#3304,.F.);
#4747=ORIENTED_EDGE('',*,*,#3297,.T.);
#4748=ORIENTED_EDGE('',*,*,#3301,.T.);
#4749=ORIENTED_EDGE('',*,*,#3309,.F.);
#4750=ORIENTED_EDGE('',*,*,#3319,.F.);
#4751=ORIENTED_EDGE('',*,*,#3313,.T.);
#4752=ORIENTED_EDGE('',*,*,#3317,.T.);
#4753=ORIENTED_EDGE('',*,*,#3066,.F.);
#4754=ORIENTED_EDGE('',*,*,#3060,.F.);
#4755=ORIENTED_EDGE('',*,*,#3053,.T.);
#4756=ORIENTED_EDGE('',*,*,#3057,.T.);
#4757=ORIENTED_EDGE('',*,*,#3065,.F.);
#4758=ORIENTED_EDGE('',*,*,#3076,.F.);
#4759=ORIENTED_EDGE('',*,*,#3069,.T.);
#4760=ORIENTED_EDGE('',*,*,#3073,.T.);
#4761=ORIENTED_EDGE('',*,*,#3080,.F.);
#4762=ORIENTED_EDGE('',*,*,#3088,.F.);
#4763=ORIENTED_EDGE('',*,*,#3081,.T.);
#4764=ORIENTED_EDGE('',*,*,#3085,.T.);
#4765=ORIENTED_EDGE('',*,*,#3092,.F.);
#4766=ORIENTED_EDGE('',*,*,#3100,.F.);
#4767=ORIENTED_EDGE('',*,*,#3093,.T.);
#4768=ORIENTED_EDGE('',*,*,#3097,.T.);
#4769=ORIENTED_EDGE('',*,*,#3104,.F.);
#4770=ORIENTED_EDGE('',*,*,#3112,.F.);
#4771=ORIENTED_EDGE('',*,*,#3105,.T.);
#4772=ORIENTED_EDGE('',*,*,#3109,.T.);
#4773=ORIENTED_EDGE('',*,*,#3116,.F.);
#4774=ORIENTED_EDGE('',*,*,#3139,.F.);
#4775=ORIENTED_EDGE('',*,*,#3133,.T.);
#4776=ORIENTED_EDGE('',*,*,#3137,.T.);
#4777=ORIENTED_EDGE('',*,*,#3130,.F.);
#4778=ORIENTED_EDGE('',*,*,#3124,.F.);
#4779=ORIENTED_EDGE('',*,*,#3117,.T.);
#4780=ORIENTED_EDGE('',*,*,#3121,.T.);
#4781=ORIENTED_EDGE('',*,*,#3129,.F.);
#4782=ORIENTED_EDGE('',*,*,#3148,.F.);
#4783=ORIENTED_EDGE('',*,*,#3141,.T.);
#4784=ORIENTED_EDGE('',*,*,#3145,.T.);
#4785=ORIENTED_EDGE('',*,*,#3152,.F.);
#4786=ORIENTED_EDGE('',*,*,#3199,.F.);
#4787=ORIENTED_EDGE('',*,*,#3193,.T.);
#4788=ORIENTED_EDGE('',*,*,#3197,.T.);
#4789=ORIENTED_EDGE('',*,*,#3166,.F.);
#4790=ORIENTED_EDGE('',*,*,#3160,.F.);
#4791=ORIENTED_EDGE('',*,*,#3153,.T.);
#4792=ORIENTED_EDGE('',*,*,#3157,.T.);
#4793=ORIENTED_EDGE('',*,*,#3165,.F.);
#4794=ORIENTED_EDGE('',*,*,#3191,.F.);
#4795=ORIENTED_EDGE('',*,*,#3185,.T.);
#4796=ORIENTED_EDGE('',*,*,#3189,.T.);
#4797=ORIENTED_EDGE('',*,*,#3182,.F.);
#4798=ORIENTED_EDGE('',*,*,#3176,.F.);
#4799=ORIENTED_EDGE('',*,*,#3169,.T.);
#4800=ORIENTED_EDGE('',*,*,#3173,.T.);
#4801=ORIENTED_EDGE('',*,*,#3181,.F.);
#4802=ORIENTED_EDGE('',*,*,#3208,.F.);
#4803=ORIENTED_EDGE('',*,*,#3201,.T.);
#4804=ORIENTED_EDGE('',*,*,#3205,.T.);
#4805=ORIENTED_EDGE('',*,*,#3212,.F.);
#4806=ORIENTED_EDGE('',*,*,#3220,.F.);
#4807=ORIENTED_EDGE('',*,*,#3213,.T.);
#4808=ORIENTED_EDGE('',*,*,#3217,.T.);
#4809=ORIENTED_EDGE('',*,*,#3224,.F.);
#4810=ORIENTED_EDGE('',*,*,#3248,.F.);
#4811=ORIENTED_EDGE('',*,*,#3241,.T.);
#4812=ORIENTED_EDGE('',*,*,#3245,.T.);
#4813=ORIENTED_EDGE('',*,*,#3252,.F.);
#4814=ORIENTED_EDGE('',*,*,#3260,.F.);
#4815=ORIENTED_EDGE('',*,*,#3253,.T.);
#4816=ORIENTED_EDGE('',*,*,#3257,.T.);
#4817=ORIENTED_EDGE('',*,*,#3264,.F.);
#4818=ORIENTED_EDGE('',*,*,#3271,.F.);
#4819=ORIENTED_EDGE('',*,*,#3265,.T.);
#4820=ORIENTED_EDGE('',*,*,#3269,.T.);
#4821=ORIENTED_EDGE('',*,*,#3238,.F.);
#4822=ORIENTED_EDGE('',*,*,#3232,.F.);
#4823=ORIENTED_EDGE('',*,*,#3225,.T.);
#4824=ORIENTED_EDGE('',*,*,#3229,.T.);
#4825=ORIENTED_EDGE('',*,*,#3237,.F.);
#4826=ORIENTED_EDGE('',*,*,#3295,.F.);
#4827=ORIENTED_EDGE('',*,*,#3289,.T.);
#4828=ORIENTED_EDGE('',*,*,#3293,.T.);
#4829=ORIENTED_EDGE('',*,*,#3286,.F.);
#4830=ORIENTED_EDGE('',*,*,#3280,.F.);
#4831=ORIENTED_EDGE('',*,*,#3273,.T.);
#4832=ORIENTED_EDGE('',*,*,#3277,.T.);
#4833=ORIENTED_EDGE('',*,*,#3285,.F.);
#4834=ORIENTED_EDGE('',*,*,#3403,.F.);
#4835=ORIENTED_EDGE('',*,*,#3397,.T.);
#4836=ORIENTED_EDGE('',*,*,#3401,.T.);
#4837=ORIENTED_EDGE('',*,*,#3386,.F.);
#4838=ORIENTED_EDGE('',*,*,#3380,.F.);
#4839=ORIENTED_EDGE('',*,*,#3373,.T.);
#4840=ORIENTED_EDGE('',*,*,#3377,.T.);
#4841=ORIENTED_EDGE('',*,*,#3385,.F.);
#4842=ORIENTED_EDGE('',*,*,#3395,.F.);
#4843=ORIENTED_EDGE('',*,*,#3389,.T.);
#4844=ORIENTED_EDGE('',*,*,#3393,.T.);
#4845=ORIENTED_EDGE('',*,*,#3370,.F.);
#4846=ORIENTED_EDGE('',*,*,#3367,.F.);
#4847=ORIENTED_EDGE('',*,*,#3361,.T.);
#4848=ORIENTED_EDGE('',*,*,#3365,.T.);
#4849=ORIENTED_EDGE('',*,*,#3334,.F.);
#4850=ORIENTED_EDGE('',*,*,#3328,.F.);
#4851=ORIENTED_EDGE('',*,*,#3321,.T.);
#4852=ORIENTED_EDGE('',*,*,#3325,.T.);
#4853=ORIENTED_EDGE('',*,*,#3333,.F.);
#4854=ORIENTED_EDGE('',*,*,#3344,.F.);
#4855=ORIENTED_EDGE('',*,*,#3337,.T.);
#4856=ORIENTED_EDGE('',*,*,#3341,.T.);
#4857=ORIENTED_EDGE('',*,*,#3348,.F.);
#4858=ORIENTED_EDGE('',*,*,#3356,.F.);
#4859=ORIENTED_EDGE('',*,*,#3349,.T.);
#4860=ORIENTED_EDGE('',*,*,#3353,.T.);
#4861=ORIENTED_EDGE('',*,*,#3423,.F.);
#4862=ORIENTED_EDGE('',*,*,#3483,.F.);
#4863=ORIENTED_EDGE('',*,*,#3430,.F.);
#4864=ORIENTED_EDGE('',*,*,#3413,.T.);
#4865=ORIENTED_EDGE('',*,*,#3417,.F.);
#4866=ORIENTED_EDGE('',*,*,#3429,.F.);
#4867=ORIENTED_EDGE('',*,*,#3433,.T.);
#4868=ORIENTED_EDGE('',*,*,#3424,.F.);
#4869=ORIENTED_EDGE('',*,*,#3435,.F.);
#4870=ORIENTED_EDGE('',*,*,#3444,.F.);
#4871=ORIENTED_EDGE('',*,*,#3445,.T.);
#4872=ORIENTED_EDGE('',*,*,#3439,.F.);
#4873=ORIENTED_EDGE('',*,*,#3447,.F.);
#4874=ORIENTED_EDGE('',*,*,#3456,.F.);
#4875=ORIENTED_EDGE('',*,*,#3457,.T.);
#4876=ORIENTED_EDGE('',*,*,#3451,.F.);
#4877=ORIENTED_EDGE('',*,*,#3459,.F.);
#4878=ORIENTED_EDGE('',*,*,#3468,.F.);
#4879=ORIENTED_EDGE('',*,*,#3469,.T.);
#4880=ORIENTED_EDGE('',*,*,#3463,.F.);
#4881=ORIENTED_EDGE('',*,*,#3485,.F.);
#4882=ORIENTED_EDGE('',*,*,#3471,.F.);
#4883=ORIENTED_EDGE('',*,*,#3480,.F.);
#4884=ORIENTED_EDGE('',*,*,#3481,.T.);
#4885=ORIENTED_EDGE('',*,*,#3475,.F.);
#5225=CYLINDRICAL_SURFACE('',#5952,25.5);
#5226=CYLINDRICAL_SURFACE('',#5955,25.5);
#5227=CYLINDRICAL_SURFACE('',#5961,25.5);
#5228=CYLINDRICAL_SURFACE('',#5967,25.5);
#5229=CYLINDRICAL_SURFACE('',#5973,25.5);
#5230=CYLINDRICAL_SURFACE('',#5979,25.5);
#5231=CYLINDRICAL_SURFACE('',#5985,25.5);
#5232=CYLINDRICAL_SURFACE('',#5988,25.5);
#5233=CYLINDRICAL_SURFACE('',#5997,25.5);
#5234=CYLINDRICAL_SURFACE('',#6003,25.5);
#5235=CYLINDRICAL_SURFACE('',#6006,25.5);
#5236=CYLINDRICAL_SURFACE('',#6012,25.5);
#5237=CYLINDRICAL_SURFACE('',#6015,25.5);
#5238=CYLINDRICAL_SURFACE('',#6027,25.5);
#5239=CYLINDRICAL_SURFACE('',#6033,25.5);
#5240=CYLINDRICAL_SURFACE('',#6039,25.5);
#5241=CYLINDRICAL_SURFACE('',#6042,25.5);
#5242=CYLINDRICAL_SURFACE('',#6048,25.5);
#5243=CYLINDRICAL_SURFACE('',#6054,25.5);
#5244=CYLINDRICAL_SURFACE('',#6063,25.5);
#5245=CYLINDRICAL_SURFACE('',#6066,25.5);
#5246=CYLINDRICAL_SURFACE('',#6075,25.5);
#5247=CYLINDRICAL_SURFACE('',#6078,25.5);
#5248=CYLINDRICAL_SURFACE('',#6087,25.5);
#5249=CYLINDRICAL_SURFACE('',#6090,25.5);
#5250=CYLINDRICAL_SURFACE('',#6096,25.5);
#5251=CYLINDRICAL_SURFACE('',#6102,25.5);
#5252=CYLINDRICAL_SURFACE('',#6108,25.5);
#5253=CYLINDRICAL_SURFACE('',#6114,25.5);
#5254=CYLINDRICAL_SURFACE('',#6117,25.5);
#5255=CYLINDRICAL_SURFACE('',#6131,22.);
#5256=CYLINDRICAL_SURFACE('',#6134,22.);
#5257=CYLINDRICAL_SURFACE('',#6137,7.00000000000001);
#5258=CYLINDRICAL_SURFACE('',#6140,7.00000000000001);
#5259=CYLINDRICAL_SURFACE('',#6145,22.);
#5260=CYLINDRICAL_SURFACE('',#6148,7.00000000000001);
#5261=CYLINDRICAL_SURFACE('',#6153,22.);
#5262=CYLINDRICAL_SURFACE('',#6156,7.00000000000001);
#5263=CYLINDRICAL_SURFACE('',#6161,22.);
#5264=CYLINDRICAL_SURFACE('',#6164,7.00000000000001);
#5265=CYLINDRICAL_SURFACE('',#6169,22.);
#5266=CYLINDRICAL_SURFACE('',#6172,7.00000000000001);
#5267=CYLINDRICAL_SURFACE('',#6177,6.00000000000001);
#5388=ADVANCED_FACE('',(#509),#202,.T.);
#5389=ADVANCED_FACE('',(#510),#203,.T.);
#5390=ADVANCED_FACE('',(#511),#204,.T.);
#5391=ADVANCED_FACE('',(#512),#5225,.T.);
#5392=ADVANCED_FACE('',(#513),#5226,.T.);
#5393=ADVANCED_FACE('',(#514),#205,.T.);
#5394=ADVANCED_FACE('',(#515),#206,.T.);
#5395=ADVANCED_FACE('',(#516),#207,.T.);
#5396=ADVANCED_FACE('',(#517),#5227,.T.);
#5397=ADVANCED_FACE('',(#518),#208,.T.);
#5398=ADVANCED_FACE('',(#519),#209,.T.);
#5399=ADVANCED_FACE('',(#520),#210,.T.);
#5400=ADVANCED_FACE('',(#521),#5228,.T.);
#5401=ADVANCED_FACE('',(#522),#211,.T.);
#5402=ADVANCED_FACE('',(#523),#212,.T.);
#5403=ADVANCED_FACE('',(#524),#213,.T.);
#5404=ADVANCED_FACE('',(#525),#5229,.T.);
#5405=ADVANCED_FACE('',(#526),#214,.T.);
#5406=ADVANCED_FACE('',(#527),#215,.T.);
#5407=ADVANCED_FACE('',(#528),#216,.T.);
#5408=ADVANCED_FACE('',(#529),#5230,.T.);
#5409=ADVANCED_FACE('',(#530),#217,.T.);
#5410=ADVANCED_FACE('',(#531),#218,.T.);
#5411=ADVANCED_FACE('',(#532),#219,.T.);
#5412=ADVANCED_FACE('',(#533),#5231,.T.);
#5413=ADVANCED_FACE('',(#534),#5232,.T.);
#5414=ADVANCED_FACE('',(#535),#220,.T.);
#5415=ADVANCED_FACE('',(#536),#221,.T.);
#5416=ADVANCED_FACE('',(#537),#222,.T.);
#5417=ADVANCED_FACE('',(#538),#223,.T.);
#5418=ADVANCED_FACE('',(#539),#224,.T.);
#5419=ADVANCED_FACE('',(#540),#225,.T.);
#5420=ADVANCED_FACE('',(#541),#5233,.T.);
#5421=ADVANCED_FACE('',(#542),#226,.T.);
#5422=ADVANCED_FACE('',(#543),#227,.T.);
#5423=ADVANCED_FACE('',(#544),#228,.T.);
#5424=ADVANCED_FACE('',(#545),#5234,.T.);
#5425=ADVANCED_FACE('',(#546),#5235,.T.);
#5426=ADVANCED_FACE('',(#547),#229,.T.);
#5427=ADVANCED_FACE('',(#548),#230,.T.);
#5428=ADVANCED_FACE('',(#549),#231,.T.);
#5429=ADVANCED_FACE('',(#550),#5236,.T.);
#5430=ADVANCED_FACE('',(#551),#5237,.T.);
#5431=ADVANCED_FACE('',(#552),#232,.T.);
#5432=ADVANCED_FACE('',(#553),#233,.T.);
#5433=ADVANCED_FACE('',(#554),#234,.T.);
#5434=ADVANCED_FACE('',(#555),#235,.T.);
#5435=ADVANCED_FACE('',(#556),#236,.T.);
#5436=ADVANCED_FACE('',(#557),#237,.T.);
#5437=ADVANCED_FACE('',(#558),#238,.T.);
#5438=ADVANCED_FACE('',(#559),#239,.T.);
#5439=ADVANCED_FACE('',(#560),#240,.T.);
#5440=ADVANCED_FACE('',(#561),#5238,.T.);
#5441=ADVANCED_FACE('',(#562),#241,.T.);
#5442=ADVANCED_FACE('',(#563),#242,.T.);
#5443=ADVANCED_FACE('',(#564),#243,.T.);
#5444=ADVANCED_FACE('',(#565),#5239,.T.);
#5445=ADVANCED_FACE('',(#566),#244,.T.);
#5446=ADVANCED_FACE('',(#567),#245,.T.);
#5447=ADVANCED_FACE('',(#568),#246,.T.);
#5448=ADVANCED_FACE('',(#569),#5240,.T.);
#5449=ADVANCED_FACE('',(#570),#5241,.T.);
#5450=ADVANCED_FACE('',(#571),#247,.T.);
#5451=ADVANCED_FACE('',(#572),#248,.T.);
#5452=ADVANCED_FACE('',(#573),#249,.T.);
#5453=ADVANCED_FACE('',(#574),#5242,.T.);
#5454=ADVANCED_FACE('',(#575),#250,.T.);
#5455=ADVANCED_FACE('',(#576),#251,.T.);
#5456=ADVANCED_FACE('',(#577),#252,.T.);
#5457=ADVANCED_FACE('',(#578),#5243,.T.);
#5458=ADVANCED_FACE('',(#579),#253,.T.);
#5459=ADVANCED_FACE('',(#580),#254,.T.);
#5460=ADVANCED_FACE('',(#581),#255,.T.);
#5461=ADVANCED_FACE('',(#582),#256,.T.);
#5462=ADVANCED_FACE('',(#583),#257,.T.);
#5463=ADVANCED_FACE('',(#584),#258,.T.);
#5464=ADVANCED_FACE('',(#585),#5244,.T.);
#5465=ADVANCED_FACE('',(#586),#5245,.T.);
#5466=ADVANCED_FACE('',(#587),#259,.T.);
#5467=ADVANCED_FACE('',(#588),#260,.T.);
#5468=ADVANCED_FACE('',(#589),#261,.T.);
#5469=ADVANCED_FACE('',(#590),#262,.T.);
#5470=ADVANCED_FACE('',(#591),#263,.T.);
#5471=ADVANCED_FACE('',(#592),#264,.T.);
#5472=ADVANCED_FACE('',(#593),#5246,.T.);
#5473=ADVANCED_FACE('',(#594),#5247,.T.);
#5474=ADVANCED_FACE('',(#595),#265,.T.);
#5475=ADVANCED_FACE('',(#596),#266,.T.);
#5476=ADVANCED_FACE('',(#597),#267,.T.);
#5477=ADVANCED_FACE('',(#598),#268,.T.);
#5478=ADVANCED_FACE('',(#599),#269,.T.);
#5479=ADVANCED_FACE('',(#600),#270,.T.);
#5480=ADVANCED_FACE('',(#601),#5248,.T.);
#5481=ADVANCED_FACE('',(#602),#5249,.T.);
#5482=ADVANCED_FACE('',(#603),#271,.T.);
#5483=ADVANCED_FACE('',(#604),#272,.T.);
#5484=ADVANCED_FACE('',(#605),#273,.T.);
#5485=ADVANCED_FACE('',(#606),#5250,.T.);
#5486=ADVANCED_FACE('',(#607),#274,.T.);
#5487=ADVANCED_FACE('',(#608),#275,.T.);
#5488=ADVANCED_FACE('',(#609),#276,.T.);
#5489=ADVANCED_FACE('',(#610),#5251,.T.);
#5490=ADVANCED_FACE('',(#611),#277,.T.);
#5491=ADVANCED_FACE('',(#612),#278,.T.);
#5492=ADVANCED_FACE('',(#613),#279,.T.);
#5493=ADVANCED_FACE('',(#614),#5252,.T.);
#5494=ADVANCED_FACE('',(#615),#280,.T.);
#5495=ADVANCED_FACE('',(#616),#281,.T.);
#5496=ADVANCED_FACE('',(#617),#282,.T.);
#5497=ADVANCED_FACE('',(#618),#5253,.T.);
#5498=ADVANCED_FACE('',(#619),#5254,.T.);
#5499=ADVANCED_FACE('',(#620),#283,.T.);
#5500=ADVANCED_FACE('',(#621),#284,.T.);
#5501=ADVANCED_FACE('',(#622),#285,.T.);
#5502=ADVANCED_FACE('',(#623),#286,.T.);
#5503=ADVANCED_FACE('',(#624),#287,.T.);
#5504=ADVANCED_FACE('',(#625),#288,.T.);
#5505=ADVANCED_FACE('',(#626),#289,.T.);
#5506=ADVANCED_FACE('',(#627),#290,.T.);
#5507=ADVANCED_FACE('',(#628),#291,.T.);
#5508=ADVANCED_FACE('',(#629),#292,.T.);
#5509=ADVANCED_FACE('',(#630),#293,.T.);
#5510=ADVANCED_FACE('',(#631),#5255,.F.);
#5511=ADVANCED_FACE('',(#632),#5256,.F.);
#5512=ADVANCED_FACE('',(#633),#5257,.T.);
#5513=ADVANCED_FACE('',(#634),#5258,.T.);
#5514=ADVANCED_FACE('',(#635),#294,.T.);
#5515=ADVANCED_FACE('',(#636),#295,.T.);
#5516=ADVANCED_FACE('',(#637),#5259,.F.);
#5517=ADVANCED_FACE('',(#638),#5260,.T.);
#5518=ADVANCED_FACE('',(#639),#296,.T.);
#5519=ADVANCED_FACE('',(#640),#297,.T.);
#5520=ADVANCED_FACE('',(#641),#5261,.F.);
#5521=ADVANCED_FACE('',(#642),#5262,.T.);
#5522=ADVANCED_FACE('',(#643),#298,.T.);
#5523=ADVANCED_FACE('',(#644),#299,.T.);
#5524=ADVANCED_FACE('',(#645),#5263,.F.);
#5525=ADVANCED_FACE('',(#646),#5264,.T.);
#5526=ADVANCED_FACE('',(#647),#300,.T.);
#5527=ADVANCED_FACE('',(#648),#301,.T.);
#5528=ADVANCED_FACE('',(#649),#5265,.F.);
#5529=ADVANCED_FACE('',(#650),#5266,.T.);
#5530=ADVANCED_FACE('',(#651),#302,.T.);
#5531=ADVANCED_FACE('',(#652),#303,.T.);
#5532=ADVANCED_FACE('',(#653),#5267,.F.);
#5533=ADVANCED_FACE('',(#654,#126,#127,#128,#129,#130,#131,#132),#304,.T.);
#5534=ADVANCED_FACE('',(#655,#133,#134,#135,#136,#137,#138,#139),#305,.F.);
#5624=CLOSED_SHELL('',(#5388,#5389,#5390,#5391,#5392,#5393,#5394,#5395,
#5396,#5397,#5398,#5399,#5400,#5401,#5402,#5403,#5404,#5405,#5406,#5407,
#5408,#5409,#5410,#5411,#5412,#5413,#5414,#5415,#5416,#5417,#5418,#5419,
#5420,#5421,#5422,#5423,#5424,#5425,#5426,#5427,#5428,#5429,#5430,#5431,
#5432,#5433,#5434,#5435,#5436,#5437,#5438,#5439,#5440,#5441,#5442,#5443,
#5444,#5445,#5446,#5447,#5448,#5449,#5450,#5451,#5452,#5453,#5454,#5455,
#5456,#5457,#5458,#5459,#5460,#5461,#5462,#5463,#5464,#5465,#5466,#5467,
#5468,#5469,#5470,#5471,#5472,#5473,#5474,#5475,#5476,#5477,#5478,#5479,
#5480,#5481,#5482,#5483,#5484,#5485,#5486,#5487,#5488,#5489,#5490,#5491,
#5492,#5493,#5494,#5495,#5496,#5497,#5498,#5499,#5500,#5501,#5502,#5503,
#5504,#5505,#5506,#5507,#5508,#5509,#5510,#5511,#5512,#5513,#5514,#5515,
#5516,#5517,#5518,#5519,#5520,#5521,#5522,#5523,#5524,#5525,#5526,#5527,
#5528,#5529,#5530,#5531,#5532,#5533,#5534));
#5948=AXIS2_PLACEMENT_3D('',#8652,#6884,#6885);
#5949=AXIS2_PLACEMENT_3D('',#8653,#6886,#6887);
#5950=AXIS2_PLACEMENT_3D('',#8662,#6892,#6893);
#5951=AXIS2_PLACEMENT_3D('',#8668,#6897,#6898);
#5952=AXIS2_PLACEMENT_3D('',#8674,#6902,#6903);
#5953=AXIS2_PLACEMENT_3D('',#8676,#6904,#6905);
#5954=AXIS2_PLACEMENT_3D('',#8679,#6907,#6908);
#5955=AXIS2_PLACEMENT_3D('',#8680,#6909,#6910);
#5956=AXIS2_PLACEMENT_3D('',#8682,#6911,#6912);
#5957=AXIS2_PLACEMENT_3D('',#8685,#6914,#6915);
#5958=AXIS2_PLACEMENT_3D('',#8686,#6916,#6917);
#5959=AXIS2_PLACEMENT_3D('',#8695,#6922,#6923);
#5960=AXIS2_PLACEMENT_3D('',#8701,#6927,#6928);
#5961=AXIS2_PLACEMENT_3D('',#8704,#6931,#6932);
#5962=AXIS2_PLACEMENT_3D('',#8706,#6933,#6934);
#5963=AXIS2_PLACEMENT_3D('',#8709,#6936,#6937);
#5964=AXIS2_PLACEMENT_3D('',#8710,#6938,#6939);
#5965=AXIS2_PLACEMENT_3D('',#8719,#6944,#6945);
#5966=AXIS2_PLACEMENT_3D('',#8725,#6949,#6950);
#5967=AXIS2_PLACEMENT_3D('',#8728,#6953,#6954);
#5968=AXIS2_PLACEMENT_3D('',#8730,#6955,#6956);
#5969=AXIS2_PLACEMENT_3D('',#8733,#6958,#6959);
#5970=AXIS2_PLACEMENT_3D('',#8734,#6960,#6961);
#5971=AXIS2_PLACEMENT_3D('',#8743,#6966,#6967);
#5972=AXIS2_PLACEMENT_3D('',#8749,#6971,#6972);
#5973=AXIS2_PLACEMENT_3D('',#8752,#6975,#6976);
#5974=AXIS2_PLACEMENT_3D('',#8754,#6977,#6978);
#5975=AXIS2_PLACEMENT_3D('',#8757,#6980,#6981);
#5976=AXIS2_PLACEMENT_3D('',#8758,#6982,#6983);
#5977=AXIS2_PLACEMENT_3D('',#8767,#6988,#6989);
#5978=AXIS2_PLACEMENT_3D('',#8773,#6993,#6994);
#5979=AXIS2_PLACEMENT_3D('',#8776,#6997,#6998);
#5980=AXIS2_PLACEMENT_3D('',#8778,#6999,#7000);
#5981=AXIS2_PLACEMENT_3D('',#8781,#7002,#7003);
#5982=AXIS2_PLACEMENT_3D('',#8782,#7004,#7005);
#5983=AXIS2_PLACEMENT_3D('',#8791,#7010,#7011);
#5984=AXIS2_PLACEMENT_3D('',#8797,#7015,#7016);
#5985=AXIS2_PLACEMENT_3D('',#8803,#7020,#7021);
#5986=AXIS2_PLACEMENT_3D('',#8805,#7022,#7023);
#5987=AXIS2_PLACEMENT_3D('',#8808,#7025,#7026);
#5988=AXIS2_PLACEMENT_3D('',#8809,#7027,#7028);
#5989=AXIS2_PLACEMENT_3D('',#8811,#7029,#7030);
#5990=AXIS2_PLACEMENT_3D('',#8814,#7032,#7033);
#5991=AXIS2_PLACEMENT_3D('',#8815,#7034,#7035);
#5992=AXIS2_PLACEMENT_3D('',#8824,#7040,#7041);
#5993=AXIS2_PLACEMENT_3D('',#8827,#7044,#7045);
#5994=AXIS2_PLACEMENT_3D('',#8830,#7048,#7049);
#5995=AXIS2_PLACEMENT_3D('',#8839,#7054,#7055);
#5996=AXIS2_PLACEMENT_3D('',#8845,#7059,#7060);
#5997=AXIS2_PLACEMENT_3D('',#8848,#7063,#7064);
#5998=AXIS2_PLACEMENT_3D('',#8850,#7065,#7066);
#5999=AXIS2_PLACEMENT_3D('',#8853,#7068,#7069);
#6000=AXIS2_PLACEMENT_3D('',#8854,#7070,#7071);
#6001=AXIS2_PLACEMENT_3D('',#8863,#7076,#7077);
#6002=AXIS2_PLACEMENT_3D('',#8869,#7081,#7082);
#6003=AXIS2_PLACEMENT_3D('',#8875,#7086,#7087);
#6004=AXIS2_PLACEMENT_3D('',#8877,#7088,#7089);
#6005=AXIS2_PLACEMENT_3D('',#8880,#7091,#7092);
#6006=AXIS2_PLACEMENT_3D('',#8881,#7093,#7094);
#6007=AXIS2_PLACEMENT_3D('',#8883,#7095,#7096);
#6008=AXIS2_PLACEMENT_3D('',#8886,#7098,#7099);
#6009=AXIS2_PLACEMENT_3D('',#8887,#7100,#7101);
#6010=AXIS2_PLACEMENT_3D('',#8896,#7106,#7107);
#6011=AXIS2_PLACEMENT_3D('',#8902,#7111,#7112);
#6012=AXIS2_PLACEMENT_3D('',#8908,#7116,#7117);
#6013=AXIS2_PLACEMENT_3D('',#8910,#7118,#7119);
#6014=AXIS2_PLACEMENT_3D('',#8913,#7121,#7122);
#6015=AXIS2_PLACEMENT_3D('',#8914,#7123,#7124);
#6016=AXIS2_PLACEMENT_3D('',#8916,#7125,#7126);
#6017=AXIS2_PLACEMENT_3D('',#8919,#7128,#7129);
#6018=AXIS2_PLACEMENT_3D('',#8920,#7130,#7131);
#6019=AXIS2_PLACEMENT_3D('',#8929,#7136,#7137);
#6020=AXIS2_PLACEMENT_3D('',#8932,#7140,#7141);
#6021=AXIS2_PLACEMENT_3D('',#8935,#7144,#7145);
#6022=AXIS2_PLACEMENT_3D('',#8944,#7150,#7151);
#6023=AXIS2_PLACEMENT_3D('',#8947,#7154,#7155);
#6024=AXIS2_PLACEMENT_3D('',#8950,#7158,#7159);
#6025=AXIS2_PLACEMENT_3D('',#8959,#7164,#7165);
#6026=AXIS2_PLACEMENT_3D('',#8965,#7169,#7170);
#6027=AXIS2_PLACEMENT_3D('',#8968,#7173,#7174);
#6028=AXIS2_PLACEMENT_3D('',#8970,#7175,#7176);
#6029=AXIS2_PLACEMENT_3D('',#8973,#7178,#7179);
#6030=AXIS2_PLACEMENT_3D('',#8974,#7180,#7181);
#6031=AXIS2_PLACEMENT_3D('',#8983,#7186,#7187);
#6032=AXIS2_PLACEMENT_3D('',#8989,#7191,#7192);
#6033=AXIS2_PLACEMENT_3D('',#8992,#7195,#7196);
#6034=AXIS2_PLACEMENT_3D('',#8994,#7197,#7198);
#6035=AXIS2_PLACEMENT_3D('',#8997,#7200,#7201);
#6036=AXIS2_PLACEMENT_3D('',#8998,#7202,#7203);
#6037=AXIS2_PLACEMENT_3D('',#9007,#7208,#7209);
#6038=AXIS2_PLACEMENT_3D('',#9013,#7213,#7214);
#6039=AXIS2_PLACEMENT_3D('',#9019,#7218,#7219);
#6040=AXIS2_PLACEMENT_3D('',#9021,#7220,#7221);
#6041=AXIS2_PLACEMENT_3D('',#9024,#7223,#7224);
#6042=AXIS2_PLACEMENT_3D('',#9025,#7225,#7226);
#6043=AXIS2_PLACEMENT_3D('',#9027,#7227,#7228);
#6044=AXIS2_PLACEMENT_3D('',#9030,#7230,#7231);
#6045=AXIS2_PLACEMENT_3D('',#9031,#7232,#7233);
#6046=AXIS2_PLACEMENT_3D('',#9040,#7238,#7239);
#6047=AXIS2_PLACEMENT_3D('',#9046,#7243,#7244);
#6048=AXIS2_PLACEMENT_3D('',#9049,#7247,#7248);
#6049=AXIS2_PLACEMENT_3D('',#9051,#7249,#7250);
#6050=AXIS2_PLACEMENT_3D('',#9054,#7252,#7253);
#6051=AXIS2_PLACEMENT_3D('',#9055,#7254,#7255);
#6052=AXIS2_PLACEMENT_3D('',#9064,#7260,#7261);
#6053=AXIS2_PLACEMENT_3D('',#9070,#7265,#7266);
#6054=AXIS2_PLACEMENT_3D('',#9073,#7269,#7270);
#6055=AXIS2_PLACEMENT_3D('',#9075,#7271,#7272);
#6056=AXIS2_PLACEMENT_3D('',#9078,#7274,#7275);
#6057=AXIS2_PLACEMENT_3D('',#9079,#7276,#7277);
#6058=AXIS2_PLACEMENT_3D('',#9088,#7282,#7283);
#6059=AXIS2_PLACEMENT_3D('',#9091,#7286,#7287);
#6060=AXIS2_PLACEMENT_3D('',#9094,#7290,#7291);
#6061=AXIS2_PLACEMENT_3D('',#9103,#7296,#7297);
#6062=AXIS2_PLACEMENT_3D('',#9109,#7301,#7302);
#6063=AXIS2_PLACEMENT_3D('',#9115,#7306,#7307);
#6064=AXIS2_PLACEMENT_3D('',#9117,#7308,#7309);
#6065=AXIS2_PLACEMENT_3D('',#9120,#7311,#7312);
#6066=AXIS2_PLACEMENT_3D('',#9121,#7313,#7314);
#6067=AXIS2_PLACEMENT_3D('',#9123,#7315,#7316);
#6068=AXIS2_PLACEMENT_3D('',#9126,#7318,#7319);
#6069=AXIS2_PLACEMENT_3D('',#9127,#7320,#7321);
#6070=AXIS2_PLACEMENT_3D('',#9136,#7326,#7327);
#6071=AXIS2_PLACEMENT_3D('',#9139,#7330,#7331);
#6072=AXIS2_PLACEMENT_3D('',#9142,#7334,#7335);
#6073=AXIS2_PLACEMENT_3D('',#9151,#7340,#7341);
#6074=AXIS2_PLACEMENT_3D('',#9157,#7345,#7346);
#6075=AXIS2_PLACEMENT_3D('',#9163,#7350,#7351);
#6076=AXIS2_PLACEMENT_3D('',#9165,#7352,#7353);
#6077=AXIS2_PLACEMENT_3D('',#9168,#7355,#7356);
#6078=AXIS2_PLACEMENT_3D('',#9169,#7357,#7358);
#6079=AXIS2_PLACEMENT_3D('',#9171,#7359,#7360);
#6080=AXIS2_PLACEMENT_3D('',#9174,#7362,#7363);
#6081=AXIS2_PLACEMENT_3D('',#9175,#7364,#7365);
#6082=AXIS2_PLACEMENT_3D('',#9184,#7370,#7371);
#6083=AXIS2_PLACEMENT_3D('',#9187,#7374,#7375);
#6084=AXIS2_PLACEMENT_3D('',#9190,#7378,#7379);
#6085=AXIS2_PLACEMENT_3D('',#9199,#7384,#7385);
#6086=AXIS2_PLACEMENT_3D('',#9205,#7389,#7390);
#6087=AXIS2_PLACEMENT_3D('',#9211,#7394,#7395);
#6088=AXIS2_PLACEMENT_3D('',#9213,#7396,#7397);
#6089=AXIS2_PLACEMENT_3D('',#9216,#7399,#7400);
#6090=AXIS2_PLACEMENT_3D('',#9217,#7401,#7402);
#6091=AXIS2_PLACEMENT_3D('',#9219,#7403,#7404);
#6092=AXIS2_PLACEMENT_3D('',#9222,#7406,#7407);
#6093=AXIS2_PLACEMENT_3D('',#9223,#7408,#7409);
#6094=AXIS2_PLACEMENT_3D('',#9232,#7414,#7415);
#6095=AXIS2_PLACEMENT_3D('',#9238,#7419,#7420);
#6096=AXIS2_PLACEMENT_3D('',#9241,#7423,#7424);
#6097=AXIS2_PLACEMENT_3D('',#9243,#7425,#7426);
#6098=AXIS2_PLACEMENT_3D('',#9246,#7428,#7429);
#6099=AXIS2_PLACEMENT_3D('',#9247,#7430,#7431);
#6100=AXIS2_PLACEMENT_3D('',#9256,#7436,#7437);
#6101=AXIS2_PLACEMENT_3D('',#9262,#7441,#7442);
#6102=AXIS2_PLACEMENT_3D('',#9265,#7445,#7446);
#6103=AXIS2_PLACEMENT_3D('',#9267,#7447,#7448);
#6104=AXIS2_PLACEMENT_3D('',#9270,#7450,#7451);
#6105=AXIS2_PLACEMENT_3D('',#9271,#7452,#7453);
#6106=AXIS2_PLACEMENT_3D('',#9280,#7458,#7459);
#6107=AXIS2_PLACEMENT_3D('',#9283,#7462,#7463);
#6108=AXIS2_PLACEMENT_3D('',#9289,#7467,#7468);
#6109=AXIS2_PLACEMENT_3D('',#9291,#7469,#7470);
#6110=AXIS2_PLACEMENT_3D('',#9294,#7472,#7473);
#6111=AXIS2_PLACEMENT_3D('',#9295,#7474,#7475);
#6112=AXIS2_PLACEMENT_3D('',#9304,#7480,#7481);
#6113=AXIS2_PLACEMENT_3D('',#9310,#7485,#7486);
#6114=AXIS2_PLACEMENT_3D('',#9316,#7490,#7491);
#6115=AXIS2_PLACEMENT_3D('',#9318,#7492,#7493);
#6116=AXIS2_PLACEMENT_3D('',#9321,#7495,#7496);
#6117=AXIS2_PLACEMENT_3D('',#9322,#7497,#7498);
#6118=AXIS2_PLACEMENT_3D('',#9324,#7499,#7500);
#6119=AXIS2_PLACEMENT_3D('',#9327,#7502,#7503);
#6120=AXIS2_PLACEMENT_3D('',#9328,#7504,#7505);
#6121=AXIS2_PLACEMENT_3D('',#9337,#7510,#7511);
#6122=AXIS2_PLACEMENT_3D('',#9340,#7514,#7515);
#6123=AXIS2_PLACEMENT_3D('',#9343,#7518,#7519);
#6124=AXIS2_PLACEMENT_3D('',#9352,#7524,#7525);
#6125=AXIS2_PLACEMENT_3D('',#9355,#7528,#7529);
#6126=AXIS2_PLACEMENT_3D('',#9358,#7532,#7533);
#6127=AXIS2_PLACEMENT_3D('',#9367,#7538,#7539);
#6128=AXIS2_PLACEMENT_3D('',#9370,#7542,#7543);
#6129=AXIS2_PLACEMENT_3D('',#9373,#7546,#7547);
#6130=AXIS2_PLACEMENT_3D('',#9382,#7552,#7553);
#6131=AXIS2_PLACEMENT_3D('',#9391,#7558,#7559);
#6132=AXIS2_PLACEMENT_3D('',#9393,#7560,#7561);
#6133=AXIS2_PLACEMENT_3D('',#9396,#7563,#7564);
#6134=AXIS2_PLACEMENT_3D('',#9397,#7565,#7566);
#6135=AXIS2_PLACEMENT_3D('',#9399,#7567,#7568);
#6136=AXIS2_PLACEMENT_3D('',#9402,#7570,#7571);
#6137=AXIS2_PLACEMENT_3D('',#9403,#7572,#7573);
#6138=AXIS2_PLACEMENT_3D('',#9405,#7574,#7575);
#6139=AXIS2_PLACEMENT_3D('',#9408,#7577,#7578);
#6140=AXIS2_PLACEMENT_3D('',#9409,#7579,#7580);
#6141=AXIS2_PLACEMENT_3D('',#9411,#7581,#7582);
#6142=AXIS2_PLACEMENT_3D('',#9414,#7584,#7585);
#6143=AXIS2_PLACEMENT_3D('',#9415,#7586,#7587);
#6144=AXIS2_PLACEMENT_3D('',#9418,#7590,#7591);
#6145=AXIS2_PLACEMENT_3D('',#9427,#7596,#7597);
#6146=AXIS2_PLACEMENT_3D('',#9429,#7598,#7599);
#6147=AXIS2_PLACEMENT_3D('',#9432,#7601,#7602);
#6148=AXIS2_PLACEMENT_3D('',#9433,#7603,#7604);
#6149=AXIS2_PLACEMENT_3D('',#9435,#7605,#7606);
#6150=AXIS2_PLACEMENT_3D('',#9438,#7608,#7609);
#6151=AXIS2_PLACEMENT_3D('',#9439,#7610,#7611);
#6152=AXIS2_PLACEMENT_3D('',#9442,#7614,#7615);
#6153=AXIS2_PLACEMENT_3D('',#9451,#7620,#7621);
#6154=AXIS2_PLACEMENT_3D('',#9453,#7622,#7623);
#6155=AXIS2_PLACEMENT_3D('',#9456,#7625,#7626);
#6156=AXIS2_PLACEMENT_3D('',#9457,#7627,#7628);
#6157=AXIS2_PLACEMENT_3D('',#9459,#7629,#7630);
#6158=AXIS2_PLACEMENT_3D('',#9462,#7632,#7633);
#6159=AXIS2_PLACEMENT_3D('',#9463,#7634,#7635);
#6160=AXIS2_PLACEMENT_3D('',#9466,#7638,#7639);
#6161=AXIS2_PLACEMENT_3D('',#9475,#7644,#7645);
#6162=AXIS2_PLACEMENT_3D('',#9477,#7646,#7647);
#6163=AXIS2_PLACEMENT_3D('',#9480,#7649,#7650);
#6164=AXIS2_PLACEMENT_3D('',#9481,#7651,#7652);
#6165=AXIS2_PLACEMENT_3D('',#9483,#7653,#7654);
#6166=AXIS2_PLACEMENT_3D('',#9486,#7656,#7657);
#6167=AXIS2_PLACEMENT_3D('',#9487,#7658,#7659);
#6168=AXIS2_PLACEMENT_3D('',#9490,#7662,#7663);
#6169=AXIS2_PLACEMENT_3D('',#9499,#7668,#7669);
#6170=AXIS2_PLACEMENT_3D('',#9501,#7670,#7671);
#6171=AXIS2_PLACEMENT_3D('',#9504,#7673,#7674);
#6172=AXIS2_PLACEMENT_3D('',#9505,#7675,#7676);
#6173=AXIS2_PLACEMENT_3D('',#9507,#7677,#7678);
#6174=AXIS2_PLACEMENT_3D('',#9510,#7680,#7681);
#6175=AXIS2_PLACEMENT_3D('',#9511,#7682,#7683);
#6176=AXIS2_PLACEMENT_3D('',#9514,#7686,#7687);
#6177=AXIS2_PLACEMENT_3D('',#9517,#7690,#7691);
#6178=AXIS2_PLACEMENT_3D('',#9519,#7692,#7693);
#6179=AXIS2_PLACEMENT_3D('',#9522,#7695,#7696);
#6180=AXIS2_PLACEMENT_3D('',#9523,#7697,#7698);
#6181=AXIS2_PLACEMENT_3D('',#9524,#7699,#7700);
#6884=DIRECTION('axis',(0.,0.,1.));
#6885=DIRECTION('refdir',(1.,0.,0.));
#6886=DIRECTION('center_axis',(0.800546781801578,0.,0.5992702646946));
#6887=DIRECTION('ref_axis',(-0.5992702646946,0.,0.800546781801578));
#6888=DIRECTION('',(0.5992702646946,0.,-0.800546781801578));
#6889=DIRECTION('',(0.,-1.,0.));
#6890=DIRECTION('',(-0.5992702646946,0.,0.800546781801578));
#6891=DIRECTION('',(0.,-1.,0.));
#6892=DIRECTION('center_axis',(0.669128232191225,0.,-0.743146963180666));
#6893=DIRECTION('ref_axis',(0.743146963180666,0.,0.669128232191225));
#6894=DIRECTION('',(-0.743146963180666,0.,-0.669128232191225));
#6895=DIRECTION('',(0.743146963180666,0.,0.669128232191225));
#6896=DIRECTION('',(0.,-1.,0.));
#6897=DIRECTION('center_axis',(-0.490545396583828,0.,0.871415637850512));
#6898=DIRECTION('ref_axis',(-0.871415637850512,0.,-0.490545396583828));
#6899=DIRECTION('',(-0.871415637850512,0.,-0.490545396583828));
#6900=DIRECTION('',(0.,1.,0.));
#6901=DIRECTION('',(-0.871415637850512,0.,-0.490545396583828));
#6902=DIRECTION('center_axis',(0.,-1.,0.));
#6903=DIRECTION('ref_axis',(1.,0.,0.));
#6904=DIRECTION('center_axis',(0.,-1.,0.));
#6905=DIRECTION('ref_axis',(1.,0.,0.));
#6906=DIRECTION('',(0.,1.,0.));
#6907=DIRECTION('center_axis',(0.,-1.,0.));
#6908=DIRECTION('ref_axis',(1.,0.,0.));
#6909=DIRECTION('center_axis',(0.,-1.,0.));
#6910=DIRECTION('ref_axis',(1.,0.,0.));
#6911=DIRECTION('center_axis',(0.,-1.,0.));
#6912=DIRECTION('ref_axis',(1.,0.,0.));
#6913=DIRECTION('',(0.,-1.,0.));
#6914=DIRECTION('center_axis',(0.,-1.,0.));
#6915=DIRECTION('ref_axis',(1.,0.,0.));
#6916=DIRECTION('center_axis',(0.907648207883844,0.,0.419731736619053));
#6917=DIRECTION('ref_axis',(-0.419731736619053,0.,0.907648207883844));
#6918=DIRECTION('',(0.419731736619053,0.,-0.907648207883844));
#6919=DIRECTION('',(0.,-1.,0.));
#6920=DIRECTION('',(-0.419731736619053,0.,0.907648207883844));
#6921=DIRECTION('',(0.,-1.,0.));
#6922=DIRECTION('center_axis',(0.499997233260123,0.,-0.866027001156559));
#6923=DIRECTION('ref_axis',(0.866027001156559,0.,0.499997233260123));
#6924=DIRECTION('',(-0.866027001156559,0.,-0.499997233260123));
#6925=DIRECTION('',(0.866027001156559,0.,0.499997233260123));
#6926=DIRECTION('',(0.,-1.,0.));
#6927=DIRECTION('center_axis',(-0.298648304048949,0.,0.954363238232009));
#6928=DIRECTION('ref_axis',(-0.954363238232009,0.,-0.298648304048949));
#6929=DIRECTION('',(-0.954363238232009,0.,-0.298648304048948));
#6930=DIRECTION('',(-0.954363238232009,0.,-0.298648304048948));
#6931=DIRECTION('center_axis',(0.,-1.,0.));
#6932=DIRECTION('ref_axis',(1.,0.,0.));
#6933=DIRECTION('center_axis',(0.,-1.,0.));
#6934=DIRECTION('ref_axis',(1.,0.,0.));
#6935=DIRECTION('',(0.,1.,0.));
#6936=DIRECTION('center_axis',(0.,-1.,0.));
#6937=DIRECTION('ref_axis',(1.,0.,0.));
#6938=DIRECTION('center_axis',(0.975081051902262,0.,0.221848917556921));
#6939=DIRECTION('ref_axis',(-0.221848917556921,0.,0.975081051902262));
#6940=DIRECTION('',(0.221848917556921,0.,-0.975081051902262));
#6941=DIRECTION('',(0.,-1.,0.));
#6942=DIRECTION('',(-0.221848917556921,0.,0.975081051902262));
#6943=DIRECTION('',(0.,-1.,0.));
#6944=DIRECTION('center_axis',(0.309013955982637,0.,-0.951057503523294));
#6945=DIRECTION('ref_axis',(0.951057503523294,0.,0.309013955982637));
#6946=DIRECTION('',(-0.951057503523294,0.,-0.309013955982637));
#6947=DIRECTION('',(0.951057503523294,0.,0.309013955982637));
#6948=DIRECTION('',(0.,-1.,0.));
#6949=DIRECTION('center_axis',(-0.0936988475535697,0.,0.995600585559858));
#6950=DIRECTION('ref_axis',(-0.995600585559858,0.,-0.0936988475535697));
#6951=DIRECTION('',(-0.995600585559858,0.,-0.0936988475535697));
#6952=DIRECTION('',(-0.995600585559858,0.,-0.0936988475535697));
#6953=DIRECTION('center_axis',(0.,-1.,0.));
#6954=DIRECTION('ref_axis',(1.,0.,0.));
#6955=DIRECTION('center_axis',(0.,-1.,0.));
#6956=DIRECTION('ref_axis',(1.,0.,0.));
#6957=DIRECTION('',(0.,1.,0.));
#6958=DIRECTION('center_axis',(0.,-1.,0.));
#6959=DIRECTION('ref_axis',(1.,0.,0.));
#6960=DIRECTION('center_axis',(0.999898174994542,0.,0.0142702362483363));
#6961=DIRECTION('ref_axis',(-0.0142702362483363,0.,0.999898174994542));
#6962=DIRECTION('',(0.0142702362483363,0.,-0.999898174994542));
#6963=DIRECTION('',(0.,-1.,0.));
#6964=DIRECTION('',(-0.0142702362483363,0.,0.999898174994542));
#6965=DIRECTION('',(0.,-1.,0.));
#6966=DIRECTION('center_axis',(0.104525286015233,0.,-0.994522229305828));
#6967=DIRECTION('ref_axis',(0.994522229305828,0.,0.104525286015233));
#6968=DIRECTION('',(-0.994522229305828,0.,-0.104525286015233));
#6969=DIRECTION('',(0.994522229305828,0.,0.104525286015233));
#6970=DIRECTION('',(0.,-1.,0.));
#6971=DIRECTION('center_axis',(0.115345698196854,0.,0.993325409877086));
#6972=DIRECTION('ref_axis',(-0.993325409877086,0.,0.115345698196854));
#6973=DIRECTION('',(-0.993325409877086,0.,0.115345698196854));
#6974=DIRECTION('',(-0.993325409877086,0.,0.115345698196854));
#6975=DIRECTION('center_axis',(0.,-1.,0.));
#6976=DIRECTION('ref_axis',(1.,0.,0.));
#6977=DIRECTION('center_axis',(0.,-1.,0.));
#6978=DIRECTION('ref_axis',(1.,0.,0.));
#6979=DIRECTION('',(0.,1.,0.));
#6980=DIRECTION('center_axis',(0.,-1.,0.));
#6981=DIRECTION('ref_axis',(1.,0.,0.));
#6982=DIRECTION('center_axis',(0.981014949795783,0.,-0.193932122860493));
#6983=DIRECTION('ref_axis',(0.193932122860493,0.,0.981014949795783));
#6984=DIRECTION('',(-0.193932122860493,0.,-0.981014949795783));
#6985=DIRECTION('',(0.,-1.,0.));
#6986=DIRECTION('',(0.193932122860493,0.,0.981014949795783));
#6987=DIRECTION('',(0.,-1.,0.));
#6988=DIRECTION('center_axis',(-0.104531640519007,0.,-0.994521561420568));
#6989=DIRECTION('ref_axis',(0.994521561420568,0.,-0.104531640519007));
#6990=DIRECTION('',(-0.994521561420568,0.,0.104531640519007));
#6991=DIRECTION('',(0.994521561420568,0.,-0.104531640519007));
#6992=DIRECTION('',(0.,-1.,0.));
#6993=DIRECTION('center_axis',(0.319349083446007,0.,0.947637147278533));
#6994=DIRECTION('ref_axis',(-0.947637147278533,0.,0.319349083446007));
#6995=DIRECTION('',(-0.947637147278533,0.,0.319349083446007));
#6996=DIRECTION('',(-0.947637147278533,0.,0.319349083446007));
#6997=DIRECTION('center_axis',(0.,-1.,0.));
#6998=DIRECTION('ref_axis',(1.,0.,0.));
#6999=DIRECTION('center_axis',(0.,-1.,0.));
#7000=DIRECTION('ref_axis',(1.,0.,0.));
#7001=DIRECTION('',(0.,1.,0.));
#7002=DIRECTION('center_axis',(0.,-1.,0.));
#7003=DIRECTION('ref_axis',(1.,0.,0.));
#7004=DIRECTION('center_axis',(0.817322450628582,0.,-0.576180537417301));
#7005=DIRECTION('ref_axis',(0.576180537417301,0.,0.817322450628582));
#7006=DIRECTION('',(-0.576180537417301,0.,-0.817322450628582));
#7007=DIRECTION('',(0.,-1.,0.));
#7008=DIRECTION('',(0.576180537417301,0.,0.817322450628582));
#7009=DIRECTION('',(0.,-1.,0.));
#7010=DIRECTION('center_axis',(-0.500002766734773,0.,-0.86602380640348));
#7011=DIRECTION('ref_axis',(0.86602380640348,0.,-0.500002766734773));
#7012=DIRECTION('',(-0.86602380640348,0.,0.500002766734773));
#7013=DIRECTION('',(0.86602380640348,0.,-0.500002766734773));
#7014=DIRECTION('',(0.,-1.,0.));
#7015=DIRECTION('center_axis',(0.677178656722426,0.,0.735818637219533));
#7016=DIRECTION('ref_axis',(-0.735818637219533,0.,0.677178656722426));
#7017=DIRECTION('',(-0.735818637219533,0.,0.677178656722426));
#7018=DIRECTION('',(0.,1.,0.));
#7019=DIRECTION('',(-0.735818637219533,0.,0.677178656722426));
#7020=DIRECTION('center_axis',(0.,-1.,0.));
#7021=DIRECTION('ref_axis',(1.,0.,0.));
#7022=DIRECTION('center_axis',(0.,-1.,0.));
#7023=DIRECTION('ref_axis',(1.,0.,0.));
#7024=DIRECTION('',(0.,1.,0.));
#7025=DIRECTION('center_axis',(0.,-1.,0.));
#7026=DIRECTION('ref_axis',(1.,0.,0.));
#7027=DIRECTION('center_axis',(0.,-1.,0.));
#7028=DIRECTION('ref_axis',(1.,0.,0.));
#7029=DIRECTION('center_axis',(0.,-1.,0.));
#7030=DIRECTION('ref_axis',(1.,0.,0.));
#7031=DIRECTION('',(0.,-1.,0.));
#7032=DIRECTION('center_axis',(0.,-1.,0.));
#7033=DIRECTION('ref_axis',(1.,0.,0.));
#7034=DIRECTION('center_axis',(0.919256663858938,0.,-0.393658717610745));
#7035=DIRECTION('ref_axis',(0.393658717610745,0.,0.919256663858937));
#7036=DIRECTION('',(-0.393658717610745,0.,-0.919256663858937));
#7037=DIRECTION('',(0.,-1.,0.));
#7038=DIRECTION('',(0.393658717610745,0.,0.919256663858937));
#7039=DIRECTION('',(0.,-1.,0.));
#7040=DIRECTION('center_axis',(-0.309020032764104,0.,-0.951055529057306));
#7041=DIRECTION('ref_axis',(0.951055529057306,0.,-0.309020032764104));
#7042=DIRECTION('',(-0.951055529057306,0.,0.309020032764104));
#7043=DIRECTION('',(0.951055529057306,0.,-0.309020032764104));
#7044=DIRECTION('center_axis',(0.50939538134165,0.,0.860532594076363));
#7045=DIRECTION('ref_axis',(-0.860532594076363,0.,0.50939538134165));
#7046=DIRECTION('',(-0.860532594076363,0.,0.50939538134165));
#7047=DIRECTION('',(-0.860532594076363,0.,0.50939538134165));
#7048=DIRECTION('center_axis',(0.679667324357505,0.,-0.733520502917751));
#7049=DIRECTION('ref_axis',(0.733520502917751,0.,0.679667324357505));
#7050=DIRECTION('',(-0.733520502917751,0.,-0.679667324357505));
#7051=DIRECTION('',(0.,-1.,0.));
#7052=DIRECTION('',(0.733520502917751,0.,0.679667324357505));
#7053=DIRECTION('',(0.,-1.,0.));
#7054=DIRECTION('center_axis',(-0.669132980519663,0.,-0.743142687766537));
#7055=DIRECTION('ref_axis',(0.743142687766537,0.,-0.669132980519663));
#7056=DIRECTION('',(-0.743142687766537,0.,0.669132980519663));
#7057=DIRECTION('',(0.743142687766537,0.,-0.669132980519663));
#7058=DIRECTION('',(0.,-1.,0.));
#7059=DIRECTION('center_axis',(0.815365975340715,0.,0.578945875066646));
#7060=DIRECTION('ref_axis',(-0.578945875066646,0.,0.815365975340715));
#7061=DIRECTION('',(-0.578945875066646,0.,0.815365975340715));
#7062=DIRECTION('',(-0.578945875066646,0.,0.815365975340715));
#7063=DIRECTION('center_axis',(0.,-1.,0.));
#7064=DIRECTION('ref_axis',(1.,0.,0.));
#7065=DIRECTION('center_axis',(0.,-1.,0.));
#7066=DIRECTION('ref_axis',(1.,0.,0.));
#7067=DIRECTION('',(0.,1.,0.));
#7068=DIRECTION('center_axis',(0.,-1.,0.));
#7069=DIRECTION('ref_axis',(1.,0.,0.));
#7070=DIRECTION('center_axis',(0.32255732989086,0.,-0.94654992944571));
#7071=DIRECTION('ref_axis',(0.94654992944571,0.,0.32255732989086));
#7072=DIRECTION('',(-0.94654992944571,0.,-0.32255732989086));
#7073=DIRECTION('',(0.,-1.,0.));
#7074=DIRECTION('',(0.94654992944571,0.,0.32255732989086));
#7075=DIRECTION('',(0.,-1.,0.));
#7076=DIRECTION('center_axis',(-0.913546757061081,0.,-0.406733724521562));
#7077=DIRECTION('ref_axis',(0.406733724521562,0.,-0.913546757061081));
#7078=DIRECTION('',(-0.406733724521561,0.,0.913546757061082));
#7079=DIRECTION('',(0.406733724521561,0.,-0.913546757061082));
#7080=DIRECTION('',(0.,-1.,0.));
#7081=DIRECTION('center_axis',(0.980352384836028,0.,0.197254154699748));
#7082=DIRECTION('ref_axis',(-0.197254154699748,0.,0.980352384836028));
#7083=DIRECTION('',(-0.197254154699748,0.,0.980352384836028));
#7084=DIRECTION('',(0.,1.,0.));
#7085=DIRECTION('',(-0.197254154699748,0.,0.980352384836028));
#7086=DIRECTION('center_axis',(0.,-1.,0.));
#7087=DIRECTION('ref_axis',(1.,0.,0.));
#7088=DIRECTION('center_axis',(0.,-1.,0.));
#7089=DIRECTION('ref_axis',(1.,0.,0.));
#7090=DIRECTION('',(0.,1.,0.));
#7091=DIRECTION('center_axis',(0.,-1.,0.));
#7092=DIRECTION('ref_axis',(1.,0.,0.));
#7093=DIRECTION('center_axis',(0.,-1.,0.));
#7094=DIRECTION('ref_axis',(1.,0.,0.));
#7095=DIRECTION('center_axis',(0.,-1.,0.));
#7096=DIRECTION('ref_axis',(1.,0.,0.));
#7097=DIRECTION('',(0.,-1.,0.));
#7098=DIRECTION('center_axis',(0.,-1.,0.));
#7099=DIRECTION('ref_axis',(1.,0.,0.));
#7100=DIRECTION('center_axis',(-0.0903257572552624,0.,-0.995912274036355));
#7101=DIRECTION('ref_axis',(0.995912274036355,0.,-0.0903257572552624));
#7102=DIRECTION('',(-0.995912274036355,0.,0.0903257572552624));
#7103=DIRECTION('',(0.,-1.,0.));
#7104=DIRECTION('',(0.995912274036355,0.,-0.0903257572552624));
#7105=DIRECTION('',(0.,-1.,0.));
#7106=DIRECTION('center_axis',(-0.999999999994897,0.,3.19475307855588E-6));
#7107=DIRECTION('ref_axis',(-3.19475307855588E-6,0.,-0.999999999994897));
#7108=DIRECTION('',(3.19475307855588E-6,0.,0.999999999994897));
#7109=DIRECTION('',(-3.19475307855588E-6,0.,-0.999999999994897));
#7110=DIRECTION('',(0.,-1.,0.));
#7111=DIRECTION('center_axis',(0.975826960771375,0.,-0.218544601012476));
#7112=DIRECTION('ref_axis',(0.218544601012476,0.,0.975826960771375));
#7113=DIRECTION('',(0.218544601012476,0.,0.975826960771374));
#7114=DIRECTION('',(0.,1.,0.));
#7115=DIRECTION('',(0.218544601012476,0.,0.975826960771374));
#7116=DIRECTION('center_axis',(0.,-1.,0.));
#7117=DIRECTION('ref_axis',(1.,0.,0.));
#7118=DIRECTION('center_axis',(0.,-1.,0.));
#7119=DIRECTION('ref_axis',(1.,0.,0.));
#7120=DIRECTION('',(0.,1.,0.));
#7121=DIRECTION('center_axis',(0.,-1.,0.));
#7122=DIRECTION('ref_axis',(1.,0.,0.));
#7123=DIRECTION('center_axis',(0.,-1.,0.));
#7124=DIRECTION('ref_axis',(1.,0.,0.));
#7125=DIRECTION('center_axis',(0.,-1.,0.));
#7126=DIRECTION('ref_axis',(1.,0.,0.));
#7127=DIRECTION('',(0.,-1.,0.));
#7128=DIRECTION('center_axis',(0.,-1.,0.));
#7129=DIRECTION('ref_axis',(1.,0.,0.));
#7130=DIRECTION('center_axis',(0.118709882057359,0.,-0.992928982305345));
#7131=DIRECTION('ref_axis',(0.992928982305345,0.,0.118709882057359));
#7132=DIRECTION('',(-0.992928982305345,0.,-0.118709882057359));
#7133=DIRECTION('',(0.,-1.,0.));
#7134=DIRECTION('',(0.992928982305345,0.,0.118709882057359));
#7135=DIRECTION('',(0.,-1.,0.));
#7136=DIRECTION('center_axis',(-0.978148264955328,0.,-0.207908565876639));
#7137=DIRECTION('ref_axis',(0.207908565876639,0.,-0.978148264955328));
#7138=DIRECTION('',(-0.207908565876639,0.,0.978148264955328));
#7139=DIRECTION('',(0.207908565876639,0.,-0.978148264955328));
#7140=DIRECTION('center_axis',(0.999940777925478,0.,-0.0108830437741485));
#7141=DIRECTION('ref_axis',(0.0108830437741485,0.,0.999940777925478));
#7142=DIRECTION('',(0.0108830437741485,0.,0.999940777925478));
#7143=DIRECTION('',(0.0108830437741485,0.,0.999940777925478));
#7144=DIRECTION('center_axis',(0.512307474606336,0.,-0.858802102618804));
#7145=DIRECTION('ref_axis',(0.858802102618804,0.,0.512307474606336));
#7146=DIRECTION('',(-0.858802102618804,0.,-0.512307474606336));
#7147=DIRECTION('',(0.,-1.,0.));
#7148=DIRECTION('',(0.858802102618804,0.,0.512307474606336));
#7149=DIRECTION('',(0.,-1.,0.));
#7150=DIRECTION('center_axis',(-0.809018872199563,0.,-0.58778266767994));
#7151=DIRECTION('ref_axis',(0.58778266767994,0.,-0.809018872199563));
#7152=DIRECTION('',(-0.58778266767994,0.,0.809018872199563));
#7153=DIRECTION('',(0.58778266767994,0.,-0.809018872199563));
#7154=DIRECTION('center_axis',(0.917917888276573,0.,0.396770400082814));
#7155=DIRECTION('ref_axis',(-0.396770400082814,0.,0.917917888276573));
#7156=DIRECTION('',(-0.396770400082814,0.,0.917917888276573));
#7157=DIRECTION('',(-0.396770400082814,0.,0.917917888276573));
#7158=DIRECTION('center_axis',(-0.295413727544757,0.,-0.955369420474673));
#7159=DIRECTION('ref_axis',(0.955369420474673,0.,-0.295413727544757));
#7160=DIRECTION('',(-0.955369420474673,0.,0.295413727544757));
#7161=DIRECTION('',(0.,-1.,0.));
#7162=DIRECTION('',(0.955369420474673,0.,-0.295413727544757));
#7163=DIRECTION('',(0.,-1.,0.));
#7164=DIRECTION('center_axis',(-0.9781469365023,0.,0.207914815756757));
#7165=DIRECTION('ref_axis',(-0.207914815756757,0.,-0.9781469365023));
#7166=DIRECTION('',(0.207914815756757,0.,0.9781469365023));
#7167=DIRECTION('',(-0.207914815756757,0.,-0.9781469365023));
#7168=DIRECTION('',(0.,-1.,0.));
#7169=DIRECTION('center_axis',(0.909064822894285,0.,-0.416654710493212));
#7170=DIRECTION('ref_axis',(0.416654710493212,0.,0.909064822894285));
#7171=DIRECTION('',(0.416654710493212,0.,0.909064822894285));
#7172=DIRECTION('',(0.416654710493212,0.,0.909064822894285));
#7173=DIRECTION('center_axis',(0.,-1.,0.));
#7174=DIRECTION('ref_axis',(1.,0.,0.));
#7175=DIRECTION('center_axis',(0.,-1.,0.));
#7176=DIRECTION('ref_axis',(1.,0.,0.));
#7177=DIRECTION('',(0.,1.,0.));
#7178=DIRECTION('center_axis',(0.,-1.,0.));
#7179=DIRECTION('ref_axis',(1.,0.,0.));
#7180=DIRECTION('center_axis',(-0.487590700388207,0.,-0.87307233886714));
#7181=DIRECTION('ref_axis',(0.87307233886714,0.,-0.487590700388207));
#7182=DIRECTION('',(-0.87307233886714,0.,0.487590700388207));
#7183=DIRECTION('',(0.,-1.,0.));
#7184=DIRECTION('',(0.87307233886714,0.,-0.487590700388207));
#7185=DIRECTION('',(0.,-1.,0.));
#7186=DIRECTION('center_axis',(-0.913544158214796,0.,0.406739561625888));
#7187=DIRECTION('ref_axis',(-0.406739561625888,0.,-0.913544158214796));
#7188=DIRECTION('',(0.406739561625888,0.,0.913544158214796));
#7189=DIRECTION('',(-0.406739561625888,0.,-0.913544158214796));
#7190=DIRECTION('',(0.,-1.,0.));
#7191=DIRECTION('center_axis',(0.802572190079719,0.,-0.596555009794272));
#7192=DIRECTION('ref_axis',(0.596555009794272,0.,0.802572190079719));
#7193=DIRECTION('',(0.596555009794272,0.,0.802572190079719));
#7194=DIRECTION('',(0.596555009794272,0.,0.802572190079719));
#7195=DIRECTION('center_axis',(0.,-1.,0.));
#7196=DIRECTION('ref_axis',(1.,0.,0.));
#7197=DIRECTION('center_axis',(0.,-1.,0.));
#7198=DIRECTION('ref_axis',(1.,0.,0.));
#7199=DIRECTION('',(0.,1.,0.));
#7200=DIRECTION('center_axis',(0.,-1.,0.));
#7201=DIRECTION('ref_axis',(1.,0.,0.));
#7202=DIRECTION('center_axis',(-0.975081051902262,0.,-0.221848917556922));
#7203=DIRECTION('ref_axis',(0.221848917556922,0.,-0.975081051902262));
#7204=DIRECTION('',(-0.221848917556922,0.,0.975081051902262));
#7205=DIRECTION('',(0.,-1.,0.));
#7206=DIRECTION('',(0.221848917556922,0.,-0.975081051902262));
#7207=DIRECTION('',(0.,-1.,0.));
#7208=DIRECTION('center_axis',(-0.309013955982637,0.,0.951057503523294));
#7209=DIRECTION('ref_axis',(-0.951057503523294,0.,-0.309013955982637));
#7210=DIRECTION('',(0.951057503523294,0.,0.309013955982637));
#7211=DIRECTION('',(-0.951057503523294,0.,-0.309013955982637));
#7212=DIRECTION('',(0.,-1.,0.));
#7213=DIRECTION('center_axis',(0.0936988475535703,0.,-0.995600585559858));
#7214=DIRECTION('ref_axis',(0.995600585559858,0.,0.0936988475535703));
#7215=DIRECTION('',(0.995600585559858,0.,0.0936988475535703));
#7216=DIRECTION('',(0.,1.,0.));
#7217=DIRECTION('',(0.995600585559858,0.,0.0936988475535703));
#7218=DIRECTION('center_axis',(0.,-1.,0.));
#7219=DIRECTION('ref_axis',(1.,0.,0.));
#7220=DIRECTION('center_axis',(0.,-1.,0.));
#7221=DIRECTION('ref_axis',(1.,0.,0.));
#7222=DIRECTION('',(0.,1.,0.));
#7223=DIRECTION('center_axis',(0.,-1.,0.));
#7224=DIRECTION('ref_axis',(1.,0.,0.));
#7225=DIRECTION('center_axis',(0.,-1.,0.));
#7226=DIRECTION('ref_axis',(1.,0.,0.));
#7227=DIRECTION('center_axis',(0.,-1.,0.));
#7228=DIRECTION('ref_axis',(1.,0.,0.));
#7229=DIRECTION('',(0.,-1.,0.));
#7230=DIRECTION('center_axis',(0.,-1.,0.));
#7231=DIRECTION('ref_axis',(1.,0.,0.));
#7232=DIRECTION('center_axis',(-0.658457619904923,0.,-0.752617806585218));
#7233=DIRECTION('ref_axis',(0.752617806585218,0.,-0.658457619904923));
#7234=DIRECTION('',(-0.752617806585218,0.,0.658457619904923));
#7235=DIRECTION('',(0.,-1.,0.));
#7236=DIRECTION('',(0.752617806585218,0.,-0.658457619904923));
#7237=DIRECTION('',(0.,-1.,0.));
#7238=DIRECTION('center_axis',(-0.809015116542074,0.,0.587787836899007));
#7239=DIRECTION('ref_axis',(-0.587787836899007,0.,-0.809015116542074));
#7240=DIRECTION('',(0.587787836899007,0.,0.809015116542074));
#7241=DIRECTION('',(-0.587787836899007,0.,-0.809015116542074));
#7242=DIRECTION('',(0.,-1.,0.));
#7243=DIRECTION('center_axis',(0.661003301390021,0.,-0.750382992578785));
#7244=DIRECTION('ref_axis',(0.750382992578785,0.,0.661003301390021));
#7245=DIRECTION('',(0.750382992578785,0.,0.661003301390021));
#7246=DIRECTION('',(0.750382992578785,0.,0.661003301390021));
#7247=DIRECTION('center_axis',(0.,-1.,0.));
#7248=DIRECTION('ref_axis',(1.,0.,0.));
#7249=DIRECTION('center_axis',(0.,-1.,0.));
#7250=DIRECTION('ref_axis',(1.,0.,0.));
#7251=DIRECTION('',(0.,1.,0.));
#7252=DIRECTION('center_axis',(0.,-1.,0.));
#7253=DIRECTION('ref_axis',(1.,0.,0.));
#7254=DIRECTION('center_axis',(-0.800546781801578,0.,-0.5992702646946));
#7255=DIRECTION('ref_axis',(0.5992702646946,0.,-0.800546781801578));
#7256=DIRECTION('',(-0.5992702646946,0.,0.800546781801578));
#7257=DIRECTION('',(0.,-1.,0.));
#7258=DIRECTION('',(0.5992702646946,0.,-0.800546781801578));
#7259=DIRECTION('',(0.,-1.,0.));
#7260=DIRECTION('center_axis',(-0.669128232191225,0.,0.743146963180666));
#7261=DIRECTION('ref_axis',(-0.743146963180666,0.,-0.669128232191225));
#7262=DIRECTION('',(0.743146963180666,0.,0.669128232191225));
#7263=DIRECTION('',(-0.743146963180666,0.,-0.669128232191225));
#7264=DIRECTION('',(0.,-1.,0.));
#7265=DIRECTION('center_axis',(0.490545396583829,0.,-0.871415637850512));
#7266=DIRECTION('ref_axis',(0.871415637850512,0.,0.490545396583829));
#7267=DIRECTION('',(0.871415637850512,0.,0.490545396583829));
#7268=DIRECTION('',(0.871415637850512,0.,0.490545396583829));
#7269=DIRECTION('center_axis',(0.,-1.,0.));
#7270=DIRECTION('ref_axis',(1.,0.,0.));
#7271=DIRECTION('center_axis',(0.,-1.,0.));
#7272=DIRECTION('ref_axis',(1.,0.,0.));
#7273=DIRECTION('',(0.,1.,0.));
#7274=DIRECTION('center_axis',(0.,-1.,0.));
#7275=DIRECTION('ref_axis',(1.,0.,0.));
#7276=DIRECTION('center_axis',(-0.907648207883844,0.,-0.419731736619053));
#7277=DIRECTION('ref_axis',(0.419731736619053,0.,-0.907648207883844));
#7278=DIRECTION('',(-0.419731736619053,0.,0.907648207883844));
#7279=DIRECTION('',(0.,-1.,0.));
#7280=DIRECTION('',(0.419731736619053,0.,-0.907648207883844));
#7281=DIRECTION('',(0.,-1.,0.));
#7282=DIRECTION('center_axis',(-0.499997233260123,0.,0.866027001156559));
#7283=DIRECTION('ref_axis',(-0.866027001156559,0.,-0.499997233260123));
#7284=DIRECTION('',(0.866027001156559,0.,0.499997233260123));
#7285=DIRECTION('',(-0.866027001156559,0.,-0.499997233260123));
#7286=DIRECTION('center_axis',(0.298648304048949,0.,-0.954363238232009));
#7287=DIRECTION('ref_axis',(0.954363238232009,0.,0.298648304048949));
#7288=DIRECTION('',(0.954363238232009,0.,0.298648304048949));
#7289=DIRECTION('',(0.954363238232009,0.,0.298648304048949));
#7290=DIRECTION('center_axis',(-0.981014949795783,0.,0.193932122860492));
#7291=DIRECTION('ref_axis',(-0.193932122860492,0.,-0.981014949795783));
#7292=DIRECTION('',(0.193932122860492,0.,0.981014949795783));
#7293=DIRECTION('',(0.,-1.,0.));
#7294=DIRECTION('',(-0.193932122860492,0.,-0.981014949795783));
#7295=DIRECTION('',(0.,-1.,0.));
#7296=DIRECTION('center_axis',(0.104531640519007,0.,0.994521561420568));
#7297=DIRECTION('ref_axis',(-0.994521561420568,0.,0.104531640519007));
#7298=DIRECTION('',(0.994521561420568,0.,-0.104531640519007));
#7299=DIRECTION('',(-0.994521561420568,0.,0.104531640519007));
#7300=DIRECTION('',(0.,-1.,0.));
#7301=DIRECTION('center_axis',(-0.319349083446007,0.,-0.947637147278533));
#7302=DIRECTION('ref_axis',(0.947637147278533,0.,-0.319349083446007));
#7303=DIRECTION('',(0.947637147278533,0.,-0.319349083446007));
#7304=DIRECTION('',(0.,1.,0.));
#7305=DIRECTION('',(0.947637147278533,0.,-0.319349083446007));
#7306=DIRECTION('center_axis',(0.,-1.,0.));
#7307=DIRECTION('ref_axis',(1.,0.,0.));
#7308=DIRECTION('center_axis',(0.,-1.,0.));
#7309=DIRECTION('ref_axis',(1.,0.,0.));
#7310=DIRECTION('',(0.,1.,0.));
#7311=DIRECTION('center_axis',(0.,-1.,0.));
#7312=DIRECTION('ref_axis',(1.,0.,0.));
#7313=DIRECTION('center_axis',(0.,-1.,0.));
#7314=DIRECTION('ref_axis',(1.,0.,0.));
#7315=DIRECTION('center_axis',(0.,-1.,0.));
#7316=DIRECTION('ref_axis',(1.,0.,0.));
#7317=DIRECTION('',(0.,-1.,0.));
#7318=DIRECTION('center_axis',(0.,-1.,0.));
#7319=DIRECTION('ref_axis',(1.,0.,0.));
#7320=DIRECTION('center_axis',(-0.999898174994542,0.,-0.0142702362483365));
#7321=DIRECTION('ref_axis',(0.0142702362483365,0.,-0.999898174994542));
#7322=DIRECTION('',(-0.0142702362483365,0.,0.999898174994542));
#7323=DIRECTION('',(0.,-1.,0.));
#7324=DIRECTION('',(0.0142702362483365,0.,-0.999898174994542));
#7325=DIRECTION('',(0.,-1.,0.));
#7326=DIRECTION('center_axis',(-0.104525286015233,0.,0.994522229305828));
#7327=DIRECTION('ref_axis',(-0.994522229305828,0.,-0.104525286015233));
#7328=DIRECTION('',(0.994522229305828,0.,0.104525286015233));
#7329=DIRECTION('',(-0.994522229305828,0.,-0.104525286015233));
#7330=DIRECTION('center_axis',(-0.115345698196854,0.,-0.993325409877086));
#7331=DIRECTION('ref_axis',(0.993325409877086,0.,-0.115345698196854));
#7332=DIRECTION('',(0.993325409877086,0.,-0.115345698196854));
#7333=DIRECTION('',(0.993325409877086,0.,-0.115345698196854));
#7334=DIRECTION('center_axis',(0.487590700388207,0.,0.87307233886714));
#7335=DIRECTION('ref_axis',(-0.87307233886714,0.,0.487590700388207));
#7336=DIRECTION('',(0.87307233886714,0.,-0.487590700388207));
#7337=DIRECTION('',(0.,-1.,0.));
#7338=DIRECTION('',(-0.87307233886714,0.,0.487590700388207));
#7339=DIRECTION('',(0.,-1.,0.));
#7340=DIRECTION('center_axis',(0.913544158214796,0.,-0.406739561625888));
#7341=DIRECTION('ref_axis',(0.406739561625888,0.,0.913544158214796));
#7342=DIRECTION('',(-0.406739561625888,0.,-0.913544158214796));
#7343=DIRECTION('',(0.406739561625888,0.,0.913544158214796));
#7344=DIRECTION('',(0.,-1.,0.));
#7345=DIRECTION('center_axis',(-0.802572190079719,0.,0.596555009794272));
#7346=DIRECTION('ref_axis',(-0.596555009794272,0.,-0.802572190079719));
#7347=DIRECTION('',(-0.596555009794272,0.,-0.802572190079719));
#7348=DIRECTION('',(0.,1.,0.));
#7349=DIRECTION('',(-0.596555009794272,0.,-0.802572190079719));
#7350=DIRECTION('center_axis',(0.,-1.,0.));
#7351=DIRECTION('ref_axis',(1.,0.,0.));
#7352=DIRECTION('center_axis',(0.,-1.,0.));
#7353=DIRECTION('ref_axis',(1.,0.,0.));
#7354=DIRECTION('',(0.,1.,0.));
#7355=DIRECTION('center_axis',(0.,-1.,0.));
#7356=DIRECTION('ref_axis',(1.,0.,0.));
#7357=DIRECTION('center_axis',(0.,-1.,0.));
#7358=DIRECTION('ref_axis',(1.,0.,0.));
#7359=DIRECTION('center_axis',(0.,-1.,0.));
#7360=DIRECTION('ref_axis',(1.,0.,0.));
#7361=DIRECTION('',(0.,-1.,0.));
#7362=DIRECTION('center_axis',(0.,-1.,0.));
#7363=DIRECTION('ref_axis',(1.,0.,0.));
#7364=DIRECTION('center_axis',(0.658457619904923,0.,0.752617806585217));
#7365=DIRECTION('ref_axis',(-0.752617806585217,0.,0.658457619904923));
#7366=DIRECTION('',(0.752617806585217,0.,-0.658457619904923));
#7367=DIRECTION('',(0.,-1.,0.));
#7368=DIRECTION('',(-0.752617806585217,0.,0.658457619904923));
#7369=DIRECTION('',(0.,-1.,0.));
#7370=DIRECTION('center_axis',(0.809015116542074,0.,-0.587787836899007));
#7371=DIRECTION('ref_axis',(0.587787836899007,0.,0.809015116542074));
#7372=DIRECTION('',(-0.587787836899007,0.,-0.809015116542074));
#7373=DIRECTION('',(0.587787836899007,0.,0.809015116542074));
#7374=DIRECTION('center_axis',(-0.661003301390021,0.,0.750382992578785));
#7375=DIRECTION('ref_axis',(-0.750382992578785,0.,-0.661003301390021));
#7376=DIRECTION('',(-0.750382992578785,0.,-0.661003301390021));
#7377=DIRECTION('',(-0.750382992578785,0.,-0.661003301390021));
#7378=DIRECTION('center_axis',(-0.32255732989086,0.,0.94654992944571));
#7379=DIRECTION('ref_axis',(-0.94654992944571,0.,-0.32255732989086));
#7380=DIRECTION('',(0.94654992944571,0.,0.32255732989086));
#7381=DIRECTION('',(0.,-1.,0.));
#7382=DIRECTION('',(-0.94654992944571,0.,-0.32255732989086));
#7383=DIRECTION('',(0.,-1.,0.));
#7384=DIRECTION('center_axis',(0.913546757061081,0.,0.406733724521562));
#7385=DIRECTION('ref_axis',(-0.406733724521562,0.,0.913546757061081));
#7386=DIRECTION('',(0.406733724521562,0.,-0.913546757061081));
#7387=DIRECTION('',(-0.406733724521562,0.,0.913546757061081));
#7388=DIRECTION('',(0.,-1.,0.));
#7389=DIRECTION('center_axis',(-0.980352384836028,0.,-0.197254154699748));
#7390=DIRECTION('ref_axis',(0.197254154699748,0.,-0.980352384836028));
#7391=DIRECTION('',(0.197254154699748,0.,-0.980352384836028));
#7392=DIRECTION('',(0.,1.,0.));
#7393=DIRECTION('',(0.197254154699748,0.,-0.980352384836028));
#7394=DIRECTION('center_axis',(0.,-1.,0.));
#7395=DIRECTION('ref_axis',(1.,0.,0.));
#7396=DIRECTION('center_axis',(0.,-1.,0.));
#7397=DIRECTION('ref_axis',(1.,0.,0.));
#7398=DIRECTION('',(0.,1.,0.));
#7399=DIRECTION('center_axis',(0.,-1.,0.));
#7400=DIRECTION('ref_axis',(1.,0.,0.));
#7401=DIRECTION('center_axis',(0.,-1.,0.));
#7402=DIRECTION('ref_axis',(1.,0.,0.));
#7403=DIRECTION('center_axis',(0.,-1.,0.));
#7404=DIRECTION('ref_axis',(1.,0.,0.));
#7405=DIRECTION('',(0.,-1.,0.));
#7406=DIRECTION('center_axis',(0.,-1.,0.));
#7407=DIRECTION('ref_axis',(1.,0.,0.));
#7408=DIRECTION('center_axis',(-0.118709882057359,0.,0.992928982305345));
#7409=DIRECTION('ref_axis',(-0.992928982305345,0.,-0.118709882057359));
#7410=DIRECTION('',(0.992928982305345,0.,0.118709882057359));
#7411=DIRECTION('',(0.,-1.,0.));
#7412=DIRECTION('',(-0.992928982305345,0.,-0.118709882057359));
#7413=DIRECTION('',(0.,-1.,0.));
#7414=DIRECTION('center_axis',(0.978148264955328,0.,0.20790856587664));
#7415=DIRECTION('ref_axis',(-0.20790856587664,0.,0.978148264955328));
#7416=DIRECTION('',(0.20790856587664,0.,-0.978148264955328));
#7417=DIRECTION('',(-0.20790856587664,0.,0.978148264955328));
#7418=DIRECTION('',(0.,-1.,0.));
#7419=DIRECTION('center_axis',(-0.999940777925478,0.,0.0108830437741482));
#7420=DIRECTION('ref_axis',(-0.0108830437741482,0.,-0.999940777925478));
#7421=DIRECTION('',(-0.0108830437741482,0.,-0.999940777925478));
#7422=DIRECTION('',(-0.0108830437741482,0.,-0.999940777925478));
#7423=DIRECTION('center_axis',(0.,-1.,0.));
#7424=DIRECTION('ref_axis',(1.,0.,0.));
#7425=DIRECTION('center_axis',(0.,-1.,0.));
#7426=DIRECTION('ref_axis',(1.,0.,0.));
#7427=DIRECTION('',(0.,1.,0.));
#7428=DIRECTION('center_axis',(0.,-1.,0.));
#7429=DIRECTION('ref_axis',(1.,0.,0.));
#7430=DIRECTION('center_axis',(0.0903257572552622,0.,0.995912274036355));
#7431=DIRECTION('ref_axis',(-0.995912274036355,0.,0.0903257572552622));
#7432=DIRECTION('',(0.995912274036355,0.,-0.0903257572552622));
#7433=DIRECTION('',(0.,-1.,0.));
#7434=DIRECTION('',(-0.995912274036355,0.,0.0903257572552622));
#7435=DIRECTION('',(0.,-1.,0.));
#7436=DIRECTION('center_axis',(0.999999999994897,0.,-3.19475307830608E-6));
#7437=DIRECTION('ref_axis',(3.19475307830608E-6,0.,0.999999999994897));
#7438=DIRECTION('',(-3.19475307830608E-6,0.,-0.999999999994897));
#7439=DIRECTION('',(3.19475307830608E-6,0.,0.999999999994897));
#7440=DIRECTION('',(0.,-1.,0.));
#7441=DIRECTION('center_axis',(-0.975826960771375,0.,0.218544601012476));
#7442=DIRECTION('ref_axis',(-0.218544601012476,0.,-0.975826960771375));
#7443=DIRECTION('',(-0.218544601012476,0.,-0.975826960771374));
#7444=DIRECTION('',(-0.218544601012476,0.,-0.975826960771374));
#7445=DIRECTION('center_axis',(0.,-1.,0.));
#7446=DIRECTION('ref_axis',(1.,0.,0.));
#7447=DIRECTION('center_axis',(0.,-1.,0.));
#7448=DIRECTION('ref_axis',(1.,0.,0.));
#7449=DIRECTION('',(0.,1.,0.));
#7450=DIRECTION('center_axis',(0.,-1.,0.));
#7451=DIRECTION('ref_axis',(1.,0.,0.));
#7452=DIRECTION('center_axis',(-0.512307474606336,0.,0.858802102618804));
#7453=DIRECTION('ref_axis',(-0.858802102618804,0.,-0.512307474606336));
#7454=DIRECTION('',(0.858802102618804,0.,0.512307474606336));
#7455=DIRECTION('',(0.,-1.,0.));
#7456=DIRECTION('',(-0.858802102618804,0.,-0.512307474606336));
#7457=DIRECTION('',(0.,-1.,0.));
#7458=DIRECTION('center_axis',(0.809018872199563,0.,0.58778266767994));
#7459=DIRECTION('ref_axis',(-0.58778266767994,0.,0.809018872199563));
#7460=DIRECTION('',(0.58778266767994,0.,-0.809018872199563));
#7461=DIRECTION('',(-0.58778266767994,0.,0.809018872199563));
#7462=DIRECTION('center_axis',(-0.917917888276573,0.,-0.396770400082814));
#7463=DIRECTION('ref_axis',(0.396770400082814,0.,-0.917917888276573));
#7464=DIRECTION('',(0.396770400082814,0.,-0.917917888276573));
#7465=DIRECTION('',(0.,1.,0.));
#7466=DIRECTION('',(0.396770400082814,0.,-0.917917888276573));
#7467=DIRECTION('center_axis',(0.,-1.,0.));
#7468=DIRECTION('ref_axis',(1.,0.,0.));
#7469=DIRECTION('center_axis',(0.,-1.,0.));
#7470=DIRECTION('ref_axis',(1.,0.,0.));
#7471=DIRECTION('',(0.,-1.,0.));
#7472=DIRECTION('center_axis',(0.,-1.,0.));
#7473=DIRECTION('ref_axis',(1.,0.,0.));
#7474=DIRECTION('center_axis',(-0.817322450628582,0.,0.576180537417301));
#7475=DIRECTION('ref_axis',(-0.576180537417301,0.,-0.817322450628582));
#7476=DIRECTION('',(0.576180537417301,0.,0.817322450628582));
#7477=DIRECTION('',(0.,-1.,0.));
#7478=DIRECTION('',(-0.576180537417301,0.,-0.817322450628582));
#7479=DIRECTION('',(0.,-1.,0.));
#7480=DIRECTION('center_axis',(0.500002766734773,0.,0.86602380640348));
#7481=DIRECTION('ref_axis',(-0.86602380640348,0.,0.500002766734773));
#7482=DIRECTION('',(0.86602380640348,0.,-0.500002766734773));
#7483=DIRECTION('',(-0.86602380640348,0.,0.500002766734773));
#7484=DIRECTION('',(0.,-1.,0.));
#7485=DIRECTION('center_axis',(-0.677178656722426,0.,-0.735818637219533));
#7486=DIRECTION('ref_axis',(0.735818637219533,0.,-0.677178656722426));
#7487=DIRECTION('',(0.735818637219533,0.,-0.677178656722426));
#7488=DIRECTION('',(0.,1.,0.));
#7489=DIRECTION('',(0.735818637219533,0.,-0.677178656722426));
#7490=DIRECTION('center_axis',(0.,-1.,0.));
#7491=DIRECTION('ref_axis',(1.,0.,0.));
#7492=DIRECTION('center_axis',(0.,-1.,0.));
#7493=DIRECTION('ref_axis',(1.,0.,0.));
#7494=DIRECTION('',(0.,1.,0.));
#7495=DIRECTION('center_axis',(0.,-1.,0.));
#7496=DIRECTION('ref_axis',(1.,0.,0.));
#7497=DIRECTION('center_axis',(0.,-1.,0.));
#7498=DIRECTION('ref_axis',(1.,0.,0.));
#7499=DIRECTION('center_axis',(0.,-1.,0.));
#7500=DIRECTION('ref_axis',(1.,0.,0.));
#7501=DIRECTION('',(0.,-1.,0.));
#7502=DIRECTION('center_axis',(0.,-1.,0.));
#7503=DIRECTION('ref_axis',(1.,0.,0.));
#7504=DIRECTION('center_axis',(-0.679667324357505,0.,0.733520502917751));
#7505=DIRECTION('ref_axis',(-0.733520502917751,0.,-0.679667324357505));
#7506=DIRECTION('',(0.733520502917751,0.,0.679667324357505));
#7507=DIRECTION('',(0.,-1.,0.));
#7508=DIRECTION('',(-0.733520502917751,0.,-0.679667324357505));
#7509=DIRECTION('',(0.,-1.,0.));
#7510=DIRECTION('center_axis',(0.669132980519662,0.,0.743142687766537));
#7511=DIRECTION('ref_axis',(-0.743142687766537,0.,0.669132980519662));
#7512=DIRECTION('',(0.743142687766537,0.,-0.669132980519662));
#7513=DIRECTION('',(-0.743142687766537,0.,0.669132980519662));
#7514=DIRECTION('center_axis',(-0.815365975340715,0.,-0.578945875066647));
#7515=DIRECTION('ref_axis',(0.578945875066647,0.,-0.815365975340715));
#7516=DIRECTION('',(0.578945875066647,0.,-0.815365975340715));
#7517=DIRECTION('',(0.578945875066647,0.,-0.815365975340715));
#7518=DIRECTION('center_axis',(-0.919256663858938,0.,0.393658717610745));
#7519=DIRECTION('ref_axis',(-0.393658717610745,0.,-0.919256663858938));
#7520=DIRECTION('',(0.393658717610745,0.,0.919256663858938));
#7521=DIRECTION('',(0.,-1.,0.));
#7522=DIRECTION('',(-0.393658717610745,0.,-0.919256663858938));
#7523=DIRECTION('',(0.,-1.,0.));
#7524=DIRECTION('center_axis',(0.309020032764104,0.,0.951055529057306));
#7525=DIRECTION('ref_axis',(-0.951055529057306,0.,0.309020032764104));
#7526=DIRECTION('',(0.951055529057306,0.,-0.309020032764104));
#7527=DIRECTION('',(-0.951055529057306,0.,0.309020032764104));
#7528=DIRECTION('center_axis',(-0.50939538134165,0.,-0.860532594076364));
#7529=DIRECTION('ref_axis',(0.860532594076364,0.,-0.50939538134165));
#7530=DIRECTION('',(0.860532594076363,0.,-0.50939538134165));
#7531=DIRECTION('',(0.860532594076363,0.,-0.50939538134165));
#7532=DIRECTION('center_axis',(0.295413727544757,0.,0.955369420474673));
#7533=DIRECTION('ref_axis',(-0.955369420474673,0.,0.295413727544757));
#7534=DIRECTION('',(0.955369420474673,0.,-0.295413727544757));
#7535=DIRECTION('',(0.,-1.,0.));
#7536=DIRECTION('',(-0.955369420474673,0.,0.295413727544757));
#7537=DIRECTION('',(0.,-1.,0.));
#7538=DIRECTION('center_axis',(0.9781469365023,0.,-0.207914815756757));
#7539=DIRECTION('ref_axis',(0.207914815756757,0.,0.9781469365023));
#7540=DIRECTION('',(-0.207914815756757,0.,-0.9781469365023));
#7541=DIRECTION('',(0.207914815756757,0.,0.9781469365023));
#7542=DIRECTION('center_axis',(-0.909064822894285,0.,0.416654710493212));
#7543=DIRECTION('ref_axis',(-0.416654710493212,0.,-0.909064822894285));
#7544=DIRECTION('',(-0.416654710493212,0.,-0.909064822894285));
#7545=DIRECTION('',(-0.416654710493212,0.,-0.909064822894285));
#7546=DIRECTION('center_axis',(0.0553951891924081,0.,0.998464507638773));
#7547=DIRECTION('ref_axis',(-0.998464507638773,0.,0.0553951891924081));
#7548=DIRECTION('',(0.998464507638773,0.,-0.0553951891924081));
#7549=DIRECTION('',(0.,1.,0.));
#7550=DIRECTION('',(-0.998464507638773,0.,0.0553951891924081));
#7551=DIRECTION('',(0.,-1.,0.));
#7552=DIRECTION('center_axis',(0.0553951891924081,0.,-0.998464507638773));
#7553=DIRECTION('ref_axis',(0.998464507638773,0.,0.0553951891924081));
#7554=DIRECTION('',(0.998464507638773,0.,0.0553951891924081));
#7555=DIRECTION('',(0.,1.,0.));
#7556=DIRECTION('',(0.998464507638773,0.,0.0553951891924081));
#7557=DIRECTION('',(0.,-1.,0.));
#7558=DIRECTION('center_axis',(0.,-1.,0.));
#7559=DIRECTION('ref_axis',(1.,0.,0.));
#7560=DIRECTION('center_axis',(0.,1.,0.));
#7561=DIRECTION('ref_axis',(1.,0.,0.));
#7562=DIRECTION('',(0.,1.,0.));
#7563=DIRECTION('center_axis',(0.,1.,0.));
#7564=DIRECTION('ref_axis',(1.,0.,0.));
#7565=DIRECTION('center_axis',(0.,-1.,0.));
#7566=DIRECTION('ref_axis',(1.,0.,0.));
#7567=DIRECTION('center_axis',(0.,1.,0.));
#7568=DIRECTION('ref_axis',(1.,0.,0.));
#7569=DIRECTION('',(0.,-1.,0.));
#7570=DIRECTION('center_axis',(0.,1.,0.));
#7571=DIRECTION('ref_axis',(1.,0.,0.));
#7572=DIRECTION('center_axis',(0.,-1.,0.));
#7573=DIRECTION('ref_axis',(1.,0.,0.));
#7574=DIRECTION('center_axis',(0.,-1.,0.));
#7575=DIRECTION('ref_axis',(1.,0.,0.));
#7576=DIRECTION('',(0.,1.,0.));
#7577=DIRECTION('center_axis',(0.,-1.,0.));
#7578=DIRECTION('ref_axis',(1.,0.,0.));
#7579=DIRECTION('center_axis',(0.,-1.,0.));
#7580=DIRECTION('ref_axis',(1.,0.,0.));
#7581=DIRECTION('center_axis',(0.,-1.,0.));
#7582=DIRECTION('ref_axis',(1.,0.,0.));
#7583=DIRECTION('',(0.,-1.,0.));
#7584=DIRECTION('center_axis',(0.,-1.,0.));
#7585=DIRECTION('ref_axis',(1.,0.,0.));
#7586=DIRECTION('center_axis',(0.892393222988503,0.,0.451258612731316));
#7587=DIRECTION('ref_axis',(-0.451258612731316,0.,0.892393222988503));
#7588=DIRECTION('',(0.451258612731316,0.,-0.892393222988503));
#7589=DIRECTION('',(-0.451258612731316,0.,0.892393222988503));
#7590=DIRECTION('center_axis',(-0.836998033796095,0.,-0.547205894907457));
#7591=DIRECTION('ref_axis',(0.547205894907457,0.,-0.836998033796095));
#7592=DIRECTION('',(0.547205894907457,0.,-0.836998033796095));
#7593=DIRECTION('',(0.,1.,0.));
#7594=DIRECTION('',(0.547205894907457,0.,-0.836998033796095));
#7595=DIRECTION('',(0.,-1.,0.));
#7596=DIRECTION('center_axis',(0.,-1.,0.));
#7597=DIRECTION('ref_axis',(1.,0.,0.));
#7598=DIRECTION('center_axis',(0.,1.,0.));
#7599=DIRECTION('ref_axis',(1.,0.,0.));
#7600=DIRECTION('',(0.,-1.,0.));
#7601=DIRECTION('center_axis',(0.,1.,0.));
#7602=DIRECTION('ref_axis',(1.,0.,0.));
#7603=DIRECTION('center_axis',(0.,-1.,0.));
#7604=DIRECTION('ref_axis',(1.,0.,0.));
#7605=DIRECTION('center_axis',(0.,-1.,0.));
#7606=DIRECTION('ref_axis',(1.,0.,0.));
#7607=DIRECTION('',(0.,1.,0.));
#7608=DIRECTION('center_axis',(0.,-1.,0.));
#7609=DIRECTION('ref_axis',(1.,0.,0.));
#7610=DIRECTION('center_axis',(0.836998033796095,0.,-0.547205894907457));
#7611=DIRECTION('ref_axis',(0.547205894907457,0.,0.836998033796095));
#7612=DIRECTION('',(-0.547205894907457,0.,-0.836998033796095));
#7613=DIRECTION('',(0.547205894907457,0.,0.836998033796095));
#7614=DIRECTION('center_axis',(-0.892393222988503,0.,0.451258612731316));
#7615=DIRECTION('ref_axis',(-0.451258612731316,0.,-0.892393222988503));
#7616=DIRECTION('',(-0.451258612731316,0.,-0.892393222988503));
#7617=DIRECTION('',(0.,1.,0.));
#7618=DIRECTION('',(-0.451258612731316,0.,-0.892393222988503));
#7619=DIRECTION('',(0.,-1.,0.));
#7620=DIRECTION('center_axis',(0.,-1.,0.));
#7621=DIRECTION('ref_axis',(1.,0.,0.));
#7622=DIRECTION('center_axis',(0.,1.,0.));
#7623=DIRECTION('ref_axis',(1.,0.,0.));
#7624=DIRECTION('',(0.,-1.,0.));
#7625=DIRECTION('center_axis',(0.,1.,0.));
#7626=DIRECTION('ref_axis',(1.,0.,0.));
#7627=DIRECTION('center_axis',(0.,-1.,0.));
#7628=DIRECTION('ref_axis',(1.,0.,0.));
#7629=DIRECTION('center_axis',(0.,-1.,0.));
#7630=DIRECTION('ref_axis',(1.,0.,0.));
#7631=DIRECTION('',(0.,1.,0.));
#7632=DIRECTION('center_axis',(0.,-1.,0.));
#7633=DIRECTION('ref_axis',(1.,0.,0.));
#7634=DIRECTION('center_axis',(-0.055395189192408,0.,-0.998464507638773));
#7635=DIRECTION('ref_axis',(0.998464507638773,0.,-0.055395189192408));
#7636=DIRECTION('',(-0.998464507638773,0.,0.055395189192408));
#7637=DIRECTION('',(0.998464507638773,0.,-0.055395189192408));
#7638=DIRECTION('center_axis',(-0.0553951891924082,0.,0.998464507638773));
#7639=DIRECTION('ref_axis',(-0.998464507638773,0.,-0.0553951891924082));
#7640=DIRECTION('',(-0.998464507638773,0.,-0.0553951891924082));
#7641=DIRECTION('',(0.,1.,0.));
#7642=DIRECTION('',(-0.998464507638773,0.,-0.0553951891924082));
#7643=DIRECTION('',(0.,-1.,0.));
#7644=DIRECTION('center_axis',(0.,-1.,0.));
#7645=DIRECTION('ref_axis',(1.,0.,0.));
#7646=DIRECTION('center_axis',(0.,1.,0.));
#7647=DIRECTION('ref_axis',(1.,0.,0.));
#7648=DIRECTION('',(0.,-1.,0.));
#7649=DIRECTION('center_axis',(0.,1.,0.));
#7650=DIRECTION('ref_axis',(1.,0.,0.));
#7651=DIRECTION('center_axis',(0.,-1.,0.));
#7652=DIRECTION('ref_axis',(1.,0.,0.));
#7653=DIRECTION('center_axis',(0.,-1.,0.));
#7654=DIRECTION('ref_axis',(1.,0.,0.));
#7655=DIRECTION('',(0.,1.,0.));
#7656=DIRECTION('center_axis',(0.,-1.,0.));
#7657=DIRECTION('ref_axis',(1.,0.,0.));
#7658=DIRECTION('center_axis',(-0.892393222988503,0.,-0.451258612731316));
#7659=DIRECTION('ref_axis',(0.451258612731316,0.,-0.892393222988503));
#7660=DIRECTION('',(-0.451258612731316,0.,0.892393222988503));
#7661=DIRECTION('',(0.451258612731316,0.,-0.892393222988503));
#7662=DIRECTION('center_axis',(0.836998033796095,0.,0.547205894907458));
#7663=DIRECTION('ref_axis',(-0.547205894907458,0.,0.836998033796095));
#7664=DIRECTION('',(-0.547205894907458,0.,0.836998033796095));
#7665=DIRECTION('',(0.,1.,0.));
#7666=DIRECTION('',(-0.547205894907458,0.,0.836998033796095));
#7667=DIRECTION('',(0.,-1.,0.));
#7668=DIRECTION('center_axis',(0.,-1.,0.));
#7669=DIRECTION('ref_axis',(1.,0.,0.));
#7670=DIRECTION('center_axis',(0.,1.,0.));
#7671=DIRECTION('ref_axis',(1.,0.,0.));
#7672=DIRECTION('',(0.,-1.,0.));
#7673=DIRECTION('center_axis',(0.,1.,0.));
#7674=DIRECTION('ref_axis',(1.,0.,0.));
#7675=DIRECTION('center_axis',(0.,-1.,0.));
#7676=DIRECTION('ref_axis',(1.,0.,0.));
#7677=DIRECTION('center_axis',(0.,-1.,0.));
#7678=DIRECTION('ref_axis',(1.,0.,0.));
#7679=DIRECTION('',(0.,1.,0.));
#7680=DIRECTION('center_axis',(0.,-1.,0.));
#7681=DIRECTION('ref_axis',(1.,0.,0.));
#7682=DIRECTION('center_axis',(-0.836998033796096,0.,0.547205894907456));
#7683=DIRECTION('ref_axis',(-0.547205894907456,0.,-0.836998033796096));
#7684=DIRECTION('',(0.547205894907456,0.,0.836998033796096));
#7685=DIRECTION('',(-0.547205894907456,0.,-0.836998033796096));
#7686=DIRECTION('center_axis',(0.892393222988504,0.,-0.451258612731315));
#7687=DIRECTION('ref_axis',(0.451258612731315,0.,0.892393222988504));
#7688=DIRECTION('',(0.451258612731315,0.,0.892393222988504));
#7689=DIRECTION('',(0.451258612731315,0.,0.892393222988504));
#7690=DIRECTION('center_axis',(0.,-1.,0.));
#7691=DIRECTION('ref_axis',(1.,0.,0.));
#7692=DIRECTION('center_axis',(0.,1.,0.));
#7693=DIRECTION('ref_axis',(1.,0.,0.));
#7694=DIRECTION('',(0.,-1.,0.));
#7695=DIRECTION('center_axis',(0.,1.,0.));
#7696=DIRECTION('ref_axis',(1.,0.,0.));
#7697=DIRECTION('center_axis',(0.,-1.,0.));
#7698=DIRECTION('ref_axis',(1.,0.,0.));
#7699=DIRECTION('center_axis',(0.,-1.,0.));
#7700=DIRECTION('ref_axis',(1.,0.,0.));
#8652=CARTESIAN_POINT('',(0.,0.,0.));
#8653=CARTESIAN_POINT('Origin',(19.5922696666578,-2.,67.8541394183561));
#8654=CARTESIAN_POINT('',(19.3381754681079,-2.,68.1935760714115));
#8655=CARTESIAN_POINT('',(19.5922696666578,-2.,67.8541394183561));
#8656=CARTESIAN_POINT('',(19.3381754681079,-2.,68.1935760714115));
#8657=CARTESIAN_POINT('',(19.3381754681079,-4.,68.1935760714115));
#8658=CARTESIAN_POINT('',(19.3381754681079,-2.,68.1935760714115));
#8659=CARTESIAN_POINT('',(19.5922696666578,-4.,67.8541394183561));
#8660=CARTESIAN_POINT('',(19.3381754681079,-4.,68.1935760714115));
#8661=CARTESIAN_POINT('',(19.5922696666578,-2.,67.8541394183561));
#8662=CARTESIAN_POINT('Origin',(14.3152323211595,-2.,63.1027041772194));
#8663=CARTESIAN_POINT('',(14.3152323211595,-2.,63.1027041772194));
#8664=CARTESIAN_POINT('',(19.5922696666578,-2.,67.8541394183561));
#8665=CARTESIAN_POINT('',(14.3152323211595,-4.,63.1027041772194));
#8666=CARTESIAN_POINT('',(19.5922696666578,-4.,67.8541394183561));
#8667=CARTESIAN_POINT('',(14.3152323211594,-2.,63.1027041772194));
#8668=CARTESIAN_POINT('Origin',(19.3381754681079,-2.,68.1935760714115));
#8669=CARTESIAN_POINT('',(12.3948017935724,-2.,64.2849475767401));
#8670=CARTESIAN_POINT('',(19.3381754681079,-2.,68.1935760714115));
#8671=CARTESIAN_POINT('',(12.3948017935724,-4.,64.2849475767401));
#8672=CARTESIAN_POINT('',(12.3948017935724,-2.,64.2849475767401));
#8673=CARTESIAN_POINT('',(19.3381754681079,-4.,68.1935760714115));
#8674=CARTESIAN_POINT('Origin',(5.11429163215176E-16,-2.,42.));
#8675=CARTESIAN_POINT('',(16.7572467664191,-4.,61.2209438064143));
#8676=CARTESIAN_POINT('Origin',(5.11429163215176E-16,-4.,42.));
#8677=CARTESIAN_POINT('',(16.7572467664191,-2.,61.2209438064143));
#8678=CARTESIAN_POINT('',(16.7572467664191,-2.,61.2209438064143));
#8679=CARTESIAN_POINT('Origin',(5.11429163215176E-16,-2.,42.));
#8680=CARTESIAN_POINT('Origin',(5.11429163215176E-16,-2.,42.));
#8681=CARTESIAN_POINT('',(9.61491124257648,-2.,65.6178636162837));
#8682=CARTESIAN_POINT('Origin',(5.11429163215176E-16,-2.,42.));
#8683=CARTESIAN_POINT('',(9.61491124257648,-4.,65.6178636162837));
#8684=CARTESIAN_POINT('',(9.61491124257649,-2.,65.6178636162837));
#8685=CARTESIAN_POINT('Origin',(5.11429163215176E-16,-4.,42.));
#8686=CARTESIAN_POINT('Origin',(24.5395094084795,-2.,63.21570252775));
#8687=CARTESIAN_POINT('',(24.3615406262698,-2.,63.6005508299847));
#8688=CARTESIAN_POINT('',(24.5395094084795,-2.,63.21570252775));
#8689=CARTESIAN_POINT('',(24.3615406262698,-2.,63.6005508299847));
#8690=CARTESIAN_POINT('',(24.3615406262698,-4.,63.6005508299847));
#8691=CARTESIAN_POINT('',(24.3615406262698,-2.,63.6005508299847));
#8692=CARTESIAN_POINT('',(24.5395094084795,-4.,63.21570252775));
#8693=CARTESIAN_POINT('',(24.3615406262698,-4.,63.6005508299847));
#8694=CARTESIAN_POINT('',(24.5395094084795,-2.,63.21570252775));
#8695=CARTESIAN_POINT('Origin',(18.3899090552018,-2.,59.6652553036011));
#8696=CARTESIAN_POINT('',(18.3899090552018,-2.,59.6652553036011));
#8697=CARTESIAN_POINT('',(24.5395094084795,-2.,63.21570252775));
#8698=CARTESIAN_POINT('',(18.3899090552018,-4.,59.6652553036011));
#8699=CARTESIAN_POINT('',(24.5395094084795,-4.,63.21570252775));
#8700=CARTESIAN_POINT('',(18.3899090552018,-2.,59.6652553036011));
#8701=CARTESIAN_POINT('Origin',(24.3615406262698,-2.,63.6005508299847));
#8702=CARTESIAN_POINT('',(24.3615406262698,-2.,63.6005508299847));
#8703=CARTESIAN_POINT('',(24.3615406262698,-4.,63.6005508299847));
#8704=CARTESIAN_POINT('Origin',(5.11429163215176E-16,-2.,42.));
#8705=CARTESIAN_POINT('',(20.3873196453819,-4.,57.3168925594268));
#8706=CARTESIAN_POINT('Origin',(5.11429163215176E-16,-4.,42.));
#8707=CARTESIAN_POINT('',(20.3873196453819,-2.,57.3168925594268));
#8708=CARTESIAN_POINT('',(20.3873196453819,-2.,57.3168925594268));
#8709=CARTESIAN_POINT('Origin',(5.11429163215176E-16,-2.,42.));
#8710=CARTESIAN_POINT('Origin',(28.41425483552,-2.,57.6500376324455));
#8711=CARTESIAN_POINT('',(28.3201895594221,-2.,58.0634778663449));
#8712=CARTESIAN_POINT('',(28.41425483552,-2.,57.6500376324455));
#8713=CARTESIAN_POINT('',(28.3201895594221,-2.,58.0634778663449));
#8714=CARTESIAN_POINT('',(28.3201895594221,-4.,58.0634778663449));
#8715=CARTESIAN_POINT('',(28.3201895594221,-2.,58.0634778663449));
#8716=CARTESIAN_POINT('',(28.41425483552,-4.,57.6500376324455));
#8717=CARTESIAN_POINT('',(28.3201895594221,-4.,58.0634778663449));
#8718=CARTESIAN_POINT('',(28.41425483552,-2.,57.6500376324455));
#8719=CARTESIAN_POINT('Origin',(21.6608585189577,-2.,55.4557500059157));
#8720=CARTESIAN_POINT('',(21.6608585189577,-2.,55.4557500059157));
#8721=CARTESIAN_POINT('',(28.41425483552,-2.,57.6500376324455));
#8722=CARTESIAN_POINT('',(21.6608585189577,-4.,55.4557500059157));
#8723=CARTESIAN_POINT('',(28.41425483552,-4.,57.6500376324455));
#8724=CARTESIAN_POINT('',(21.6608585189577,-2.,55.4557500059157));
#8725=CARTESIAN_POINT('Origin',(28.3201895594221,-2.,58.0634778663449));
#8726=CARTESIAN_POINT('',(28.3201895594221,-2.,58.0634778663449));
#8727=CARTESIAN_POINT('',(28.3201895594221,-4.,58.0634778663449));
#8728=CARTESIAN_POINT('Origin',(5.11429163215176E-16,-2.,42.));
#8729=CARTESIAN_POINT('',(23.1263688266279,-4.,52.7434196089874));
#8730=CARTESIAN_POINT('Origin',(5.11429163215176E-16,-4.,42.));
#8731=CARTESIAN_POINT('',(23.1263688266279,-2.,52.7434196089874));
#8732=CARTESIAN_POINT('',(23.1263688266279,-2.,52.7434196089874));
#8733=CARTESIAN_POINT('Origin',(5.11429163215176E-16,-2.,42.));
#8734=CARTESIAN_POINT('Origin',(31.0471609795261,-2.,51.4003909953907));
#8735=CARTESIAN_POINT('',(31.0411103134807,-2.,51.8243538388269));
#8736=CARTESIAN_POINT('',(31.0471609795261,-2.,51.4003909953907));
#8737=CARTESIAN_POINT('',(31.0411103134807,-2.,51.8243538388269));
#8738=CARTESIAN_POINT('',(31.0411103134807,-4.,51.8243538388269));
#8739=CARTESIAN_POINT('',(31.0411103134807,-2.,51.8243538388269));
#8740=CARTESIAN_POINT('',(31.0471609795261,-4.,51.4003909953907));
#8741=CARTESIAN_POINT('',(31.0411103134807,-4.,51.8243538388269));
#8742=CARTESIAN_POINT('',(31.0471609795261,-2.,51.4003909953907));
#8743=CARTESIAN_POINT('Origin',(23.9851245251038,-2.,50.6581638651196));
#8744=CARTESIAN_POINT('',(23.9851245251038,-2.,50.6581638651196));
#8745=CARTESIAN_POINT('',(31.0471609795261,-2.,51.4003909953907));
#8746=CARTESIAN_POINT('',(23.9851245251038,-4.,50.6581638651196));
#8747=CARTESIAN_POINT('',(31.0471609795261,-4.,51.4003909953907));
#8748=CARTESIAN_POINT('',(23.9851245251038,-2.,50.6581638651196));
#8749=CARTESIAN_POINT('Origin',(31.0411103134807,-2.,51.8243538388269));
#8750=CARTESIAN_POINT('',(31.0411103134807,-2.,51.8243538388269));
#8751=CARTESIAN_POINT('',(31.0411103134807,-4.,51.8243538388269));
#8752=CARTESIAN_POINT('Origin',(5.11429163215176E-16,-2.,42.));
#8753=CARTESIAN_POINT('',(24.8546847175204,-4.,47.7004076689882));
#8754=CARTESIAN_POINT('Origin',(5.11429163215176E-16,-4.,42.));
#8755=CARTESIAN_POINT('',(24.8546847175204,-2.,47.7004076689882));
#8756=CARTESIAN_POINT('',(24.8546847175204,-2.,47.7004076689882));
#8757=CARTESIAN_POINT('Origin',(5.11429163215176E-16,-2.,42.));
#8758=CARTESIAN_POINT('Origin',(32.3231572079194,-2.,44.7399021637567));
#8759=CARTESIAN_POINT('',(32.405385595067,-2.,45.1558584060722));
#8760=CARTESIAN_POINT('',(32.3231572079194,-2.,44.7399021637567));
#8761=CARTESIAN_POINT('',(32.405385595067,-2.,45.1558584060722));
#8762=CARTESIAN_POINT('',(32.405385595067,-4.,45.1558584060722));
#8763=CARTESIAN_POINT('',(32.405385595067,-2.,45.1558584060722));
#8764=CARTESIAN_POINT('',(32.3231572079194,-4.,44.7399021637567));
#8765=CARTESIAN_POINT('',(32.405385595067,-4.,45.1558584060722));
#8766=CARTESIAN_POINT('',(32.3231572079194,-2.,44.7399021637567));
#8767=CARTESIAN_POINT('Origin',(25.2611254961061,-2.,45.482174416938));
#8768=CARTESIAN_POINT('',(25.2611254961061,-2.,45.482174416938));
#8769=CARTESIAN_POINT('',(32.3231572079194,-2.,44.7399021637567));
#8770=CARTESIAN_POINT('',(25.2611254961061,-4.,45.482174416938));
#8771=CARTESIAN_POINT('',(32.3231572079194,-4.,44.7399021637567));
#8772=CARTESIAN_POINT('',(25.2611254961061,-2.,45.482174416938));
#8773=CARTESIAN_POINT('Origin',(32.405385595067,-2.,45.1558584060722));
#8774=CARTESIAN_POINT('',(32.405385595067,-2.,45.1558584060722));
#8775=CARTESIAN_POINT('',(32.405385595067,-4.,45.1558584060722));
#8776=CARTESIAN_POINT('Origin',(5.11429163215176E-16,-2.,42.));
#8777=CARTESIAN_POINT('',(25.4967316202476,-4.,42.4082605602634));
#8778=CARTESIAN_POINT('Origin',(5.11429163215176E-16,-4.,42.));
#8779=CARTESIAN_POINT('',(25.4967316202476,-2.,42.4082605602634));
#8780=CARTESIAN_POINT('',(25.4967316202476,-2.,42.4082605602634));
#8781=CARTESIAN_POINT('Origin',(5.11429163215176E-16,-2.,42.));
#8782=CARTESIAN_POINT('Origin',(30.643092052405,-2.,31.3560127197245));
#8783=CARTESIAN_POINT('',(30.8873960676387,-2.,31.702562357316));
#8784=CARTESIAN_POINT('',(30.643092052405,-2.,31.3560127197245));
#8785=CARTESIAN_POINT('',(30.8873960676387,-2.,31.702562357316));
#8786=CARTESIAN_POINT('',(30.8873960676387,-4.,31.702562357316));
#8787=CARTESIAN_POINT('',(30.8873960676387,-2.,31.702562357316));
#8788=CARTESIAN_POINT('',(30.643092052405,-4.,31.3560127197245));
#8789=CARTESIAN_POINT('',(30.8873960676387,-4.,31.702562357316));
#8790=CARTESIAN_POINT('',(30.643092052405,-2.,31.3560127197245));
#8791=CARTESIAN_POINT('Origin',(24.4935143848573,-2.,34.9064992367103));
#8792=CARTESIAN_POINT('',(24.4935143848573,-2.,34.9064992367103));
#8793=CARTESIAN_POINT('',(30.643092052405,-2.,31.3560127197245));
#8794=CARTESIAN_POINT('',(24.4935143848573,-4.,34.9064992367103));
#8795=CARTESIAN_POINT('',(30.643092052405,-4.,31.3560127197245));
#8796=CARTESIAN_POINT('',(24.4935143848573,-2.,34.9064992367103));
#8797=CARTESIAN_POINT('Origin',(30.8873960676387,-2.,31.702562357316));
#8798=CARTESIAN_POINT('',(25.0244490042775,-2.,37.0982705060036));
#8799=CARTESIAN_POINT('',(30.8873960676387,-2.,31.702562357316));
#8800=CARTESIAN_POINT('',(25.0244490042775,-4.,37.0982705060036));
#8801=CARTESIAN_POINT('',(25.0244490042775,-2.,37.0982705060036));
#8802=CARTESIAN_POINT('',(30.8873960676387,-4.,31.702562357316));
#8803=CARTESIAN_POINT('Origin',(5.11429163215176E-16,-2.,42.));
#8804=CARTESIAN_POINT('',(23.4584778861915,-4.,32.0025095517392));
#8805=CARTESIAN_POINT('Origin',(5.11429163215176E-16,-4.,42.));
#8806=CARTESIAN_POINT('',(23.4584778861915,-2.,32.0025095517392));
#8807=CARTESIAN_POINT('',(23.4584778861915,-2.,32.0025095517392));
#8808=CARTESIAN_POINT('Origin',(5.11429163215176E-16,-2.,42.));
#8809=CARTESIAN_POINT('Origin',(5.11429163215176E-16,-2.,42.));
#8810=CARTESIAN_POINT('',(25.4330940665997,-2.,40.1539972374095));
#8811=CARTESIAN_POINT('Origin',(5.11429163215176E-16,-2.,42.));
#8812=CARTESIAN_POINT('',(25.4330940665997,-4.,40.1539972374095));
#8813=CARTESIAN_POINT('',(25.4330940665997,-2.,40.1539972374095));
#8814=CARTESIAN_POINT('Origin',(5.11429163215176E-16,-4.,42.));
#8815=CARTESIAN_POINT('Origin',(32.1864763626099,-2.,37.9596664600572));
#8816=CARTESIAN_POINT('',(32.3533900278565,-2.,38.3494368174833));
#8817=CARTESIAN_POINT('',(32.1864763626099,-2.,37.9596664600572));
#8818=CARTESIAN_POINT('',(32.3533900278565,-2.,38.3494368174833));
#8819=CARTESIAN_POINT('',(32.3533900278565,-4.,38.3494368174833));
#8820=CARTESIAN_POINT('',(32.3533900278565,-2.,38.3494368174833));
#8821=CARTESIAN_POINT('',(32.1864763626099,-4.,37.9596664600572));
#8822=CARTESIAN_POINT('',(32.3533900278565,-4.,38.3494368174833));
#8823=CARTESIAN_POINT('',(32.1864763626099,-2.,37.9596664600572));
#8824=CARTESIAN_POINT('Origin',(25.4330940665997,-2.,40.1539972374095));
#8825=CARTESIAN_POINT('',(32.1864763626099,-2.,37.9596664600572));
#8826=CARTESIAN_POINT('',(32.1864763626099,-4.,37.9596664600572));
#8827=CARTESIAN_POINT('Origin',(32.3533900278565,-2.,38.3494368174833));
#8828=CARTESIAN_POINT('',(32.3533900278565,-2.,38.3494368174833));
#8829=CARTESIAN_POINT('',(32.3533900278565,-4.,38.3494368174833));
#8830=CARTESIAN_POINT('Origin',(27.7604575776403,-2.,25.2175522990576));
#8831=CARTESIAN_POINT('',(28.0714746850947,-2.,25.5057353347221));
#8832=CARTESIAN_POINT('',(27.7604575776403,-2.,25.2175522990576));
#8833=CARTESIAN_POINT('',(28.0714746850947,-2.,25.5057353347221));
#8834=CARTESIAN_POINT('',(28.0714746850947,-4.,25.5057353347221));
#8835=CARTESIAN_POINT('',(28.0714746850947,-2.,25.5057353347221));
#8836=CARTESIAN_POINT('',(27.7604575776403,-4.,25.2175522990576));
#8837=CARTESIAN_POINT('',(28.0714746850947,-4.,25.5057353347221));
#8838=CARTESIAN_POINT('',(27.7604575776403,-2.,25.2175522990576));
#8839=CARTESIAN_POINT('Origin',(22.4834505915744,-2.,29.96902125776));
#8840=CARTESIAN_POINT('',(22.4834505915744,-2.,29.96902125776));
#8841=CARTESIAN_POINT('',(27.7604575776403,-2.,25.2175522990576));
#8842=CARTESIAN_POINT('',(22.4834505915744,-4.,29.96902125776));
#8843=CARTESIAN_POINT('',(27.7604575776403,-4.,25.2175522990576));
#8844=CARTESIAN_POINT('',(22.4834505915744,-2.,29.96902125776));
#8845=CARTESIAN_POINT('Origin',(28.0714746850947,-2.,25.5057353347221));
#8846=CARTESIAN_POINT('',(28.0714746850947,-2.,25.5057353347221));
#8847=CARTESIAN_POINT('',(28.0714746850947,-4.,25.5057353347221));
#8848=CARTESIAN_POINT('Origin',(5.11429163215176E-16,-2.,42.));
#8849=CARTESIAN_POINT('',(20.8672587182129,-4.,27.3436869033454));
#8850=CARTESIAN_POINT('Origin',(5.11429163215176E-16,-4.,42.));
#8851=CARTESIAN_POINT('',(20.8672587182129,-2.,27.3436869033454));
#8852=CARTESIAN_POINT('',(20.8672587182129,-2.,27.3436869033454));
#8853=CARTESIAN_POINT('Origin',(5.11429163215176E-16,-2.,42.));
#8854=CARTESIAN_POINT('Origin',(18.5344034816569,-2.,15.377275809302));
#8855=CARTESIAN_POINT('',(18.9357463479386,-2.,15.5140420582778));
#8856=CARTESIAN_POINT('',(18.5344034816569,-2.,15.377275809302));
#8857=CARTESIAN_POINT('',(18.9357463479386,-2.,15.5140420582778));
#8858=CARTESIAN_POINT('',(18.9357463479386,-4.,15.5140420582778));
#8859=CARTESIAN_POINT('',(18.9357463479386,-2.,15.5140420582778));
#8860=CARTESIAN_POINT('',(18.5344034816569,-4.,15.377275809302));
#8861=CARTESIAN_POINT('',(18.9357463479386,-4.,15.5140420582778));
#8862=CARTESIAN_POINT('',(18.5344034816569,-2.,15.377275809302));
#8863=CARTESIAN_POINT('Origin',(15.6462142535297,-2.,21.8643108006543));
#8864=CARTESIAN_POINT('',(15.6462142535297,-2.,21.8643108006543));
#8865=CARTESIAN_POINT('',(18.5344034816569,-2.,15.377275809302));
#8866=CARTESIAN_POINT('',(15.6462142535297,-4.,21.8643108006543));
#8867=CARTESIAN_POINT('',(18.5344034816569,-4.,15.377275809302));
#8868=CARTESIAN_POINT('',(15.6462142535297,-2.,21.8643108006543));
#8869=CARTESIAN_POINT('Origin',(18.9357463479386,-2.,15.5140420582778));
#8870=CARTESIAN_POINT('',(17.3640402120316,-2.,23.3254154660686));
#8871=CARTESIAN_POINT('',(18.9357463479386,-2.,15.5140420582778));
#8872=CARTESIAN_POINT('',(17.3640402120316,-4.,23.3254154660686));
#8873=CARTESIAN_POINT('',(17.3640402120316,-2.,23.3254154660686));
#8874=CARTESIAN_POINT('',(18.9357463479386,-4.,15.5140420582778));
#8875=CARTESIAN_POINT('Origin',(5.11429163215176E-16,-2.,42.));
#8876=CARTESIAN_POINT('',(13.1019298266752,-4.,20.1233129835233));
#8877=CARTESIAN_POINT('Origin',(5.11429163215176E-16,-4.,42.));
#8878=CARTESIAN_POINT('',(13.1019298266752,-2.,20.1233129835233));
#8879=CARTESIAN_POINT('',(13.1019298266752,-2.,20.1233129835233));
#8880=CARTESIAN_POINT('Origin',(5.11429163215176E-16,-2.,42.));
#8881=CARTESIAN_POINT('Origin',(5.11429163215176E-16,-2.,42.));
#8882=CARTESIAN_POINT('',(19.490752119874,-2.,25.5573547808867));
#8883=CARTESIAN_POINT('Origin',(5.11429163215176E-16,-2.,42.));
#8884=CARTESIAN_POINT('',(19.490752119874,-4.,25.5573547808867));
#8885=CARTESIAN_POINT('',(19.490752119874,-2.,25.5573547808867));
#8886=CARTESIAN_POINT('Origin',(5.11429163215176E-16,-4.,42.));
#8887=CARTESIAN_POINT('Origin',(6.1035826439255,-2.,10.1403101919745));
#8888=CARTESIAN_POINT('',(6.52585544136889,-2.,10.1020115273313));
#8889=CARTESIAN_POINT('',(6.1035826439255,-2.,10.1403101919745));
#8890=CARTESIAN_POINT('',(6.52585544136889,-2.,10.1020115273313));
#8891=CARTESIAN_POINT('',(6.52585544136889,-4.,10.1020115273313));
#8892=CARTESIAN_POINT('',(6.52585544136889,-2.,10.1020115273313));
#8893=CARTESIAN_POINT('',(6.1035826439255,-4.,10.1403101919745));
#8894=CARTESIAN_POINT('',(6.52585544136889,-4.,10.1020115273313));
#8895=CARTESIAN_POINT('',(6.1035826439255,-2.,10.1403101919745));
#8896=CARTESIAN_POINT('Origin',(6.10360532965543,-2.,17.2412439331092));
#8897=CARTESIAN_POINT('',(6.10360532965543,-2.,17.2412439331092));
#8898=CARTESIAN_POINT('',(6.1035826439255,-2.,10.1403101919745));
#8899=CARTESIAN_POINT('',(6.10360532965543,-4.,17.2412439331092));
#8900=CARTESIAN_POINT('',(6.1035826439255,-4.,10.1403101919745));
#8901=CARTESIAN_POINT('',(6.10360532965543,-2.,17.2412439331092));
#8902=CARTESIAN_POINT('Origin',(6.52585544136889,-2.,10.1020115273313));
#8903=CARTESIAN_POINT('',(8.26720223785844,-2.,17.8773266995893));
#8904=CARTESIAN_POINT('',(6.52585544136889,-2.,10.1020115273313));
#8905=CARTESIAN_POINT('',(8.26720223785844,-4.,17.8773266995893));
#8906=CARTESIAN_POINT('',(8.26720223785844,-2.,17.8773266995893));
#8907=CARTESIAN_POINT('',(6.52585544136889,-4.,10.1020115273313));
#8908=CARTESIAN_POINT('Origin',(5.11429163215176E-16,-2.,42.));
#8909=CARTESIAN_POINT('',(3.07115824080957,-4.,16.6856169923123));
#8910=CARTESIAN_POINT('Origin',(5.11429163215176E-16,-4.,42.));
#8911=CARTESIAN_POINT('',(3.07115824080957,-2.,16.6856169923123));
#8912=CARTESIAN_POINT('',(3.07115824080957,-2.,16.6856169923123));
#8913=CARTESIAN_POINT('Origin',(5.11429163215176E-16,-2.,42.));
#8914=CARTESIAN_POINT('Origin',(5.11429163215176E-16,-2.,42.));
#8915=CARTESIAN_POINT('',(11.1178617454402,-2.,19.0512930601901));
#8916=CARTESIAN_POINT('Origin',(5.11429163215176E-16,-2.,42.));
#8917=CARTESIAN_POINT('',(11.1178617454402,-4.,19.0512930601901));
#8918=CARTESIAN_POINT('',(11.1178617454402,-2.,19.0512930601901));
#8919=CARTESIAN_POINT('Origin',(5.11429163215176E-16,-4.,42.));
#8920=CARTESIAN_POINT('Origin',(12.5942066959521,-2.,12.1055270417011));
#8921=CARTESIAN_POINT('',(13.0152145597486,-2.,12.1558607460718));
#8922=CARTESIAN_POINT('',(12.5942066959521,-2.,12.1055270417011));
#8923=CARTESIAN_POINT('',(13.0152145597486,-2.,12.1558607460718));
#8924=CARTESIAN_POINT('',(13.0152145597486,-4.,12.1558607460718));
#8925=CARTESIAN_POINT('',(13.0152145597486,-2.,12.1558607460718));
#8926=CARTESIAN_POINT('',(12.5942066959521,-4.,12.1055270417011));
#8927=CARTESIAN_POINT('',(13.0152145597486,-4.,12.1558607460718));
#8928=CARTESIAN_POINT('',(12.5942066959521,-2.,12.1055270417011));
#8929=CARTESIAN_POINT('Origin',(11.1178617454402,-2.,19.0512930601901));
#8930=CARTESIAN_POINT('',(12.5942066959521,-2.,12.1055270417011));
#8931=CARTESIAN_POINT('',(12.5942066959521,-4.,12.1055270417011));
#8932=CARTESIAN_POINT('Origin',(13.0152145597486,-2.,12.1558607460718));
#8933=CARTESIAN_POINT('',(13.0152145597486,-2.,12.1558607460718));
#8934=CARTESIAN_POINT('',(13.0152145597486,-4.,12.1558607460718));
#8935=CARTESIAN_POINT('Origin',(23.6645578972779,-2.,19.8125653740408));
#8936=CARTESIAN_POINT('',(24.0286951569316,-2.,20.0297868262641));
#8937=CARTESIAN_POINT('',(23.6645578972779,-2.,19.8125653740408));
#8938=CARTESIAN_POINT('',(24.0286951569316,-2.,20.0297868262641));
#8939=CARTESIAN_POINT('',(24.0286951569316,-4.,20.0297868262641));
#8940=CARTESIAN_POINT('',(24.0286951569316,-2.,20.0297868262641));
#8941=CARTESIAN_POINT('',(23.6645578972779,-4.,19.8125653740408));
#8942=CARTESIAN_POINT('',(24.0286951569316,-4.,20.0297868262641));
#8943=CARTESIAN_POINT('',(23.6645578972779,-2.,19.8125653740408));
#8944=CARTESIAN_POINT('Origin',(19.490752119874,-2.,25.5573547808867));
#8945=CARTESIAN_POINT('',(23.6645578972779,-2.,19.8125653740408));
#8946=CARTESIAN_POINT('',(23.6645578972779,-4.,19.8125653740408));
#8947=CARTESIAN_POINT('Origin',(24.0286951569316,-2.,20.0297868262641));
#8948=CARTESIAN_POINT('',(24.0286951569316,-2.,20.0297868262641));
#8949=CARTESIAN_POINT('',(24.0286951569316,-4.,20.0297868262641));
#8950=CARTESIAN_POINT('Origin',(-0.653797257879687,-2.,9.5675146666121));
#8951=CARTESIAN_POINT('',(-0.248714874327312,-2.,9.44225746837724));
#8952=CARTESIAN_POINT('',(-0.653797257879687,-2.,9.5675146666121));
#8953=CARTESIAN_POINT('',(-0.248714874327312,-2.,9.44225746837724));
#8954=CARTESIAN_POINT('',(-0.248714874327312,-4.,9.44225746837724));
#8955=CARTESIAN_POINT('',(-0.248714874327312,-2.,9.44225746837724));
#8956=CARTESIAN_POINT('',(-0.653797257879687,-4.,9.5675146666121));
#8957=CARTESIAN_POINT('',(-0.248714874327312,-4.,9.44225746837724));
#8958=CARTESIAN_POINT('',(-0.653797257879687,-2.,9.5675146666121));
#8959=CARTESIAN_POINT('Origin',(0.822592072616804,-2.,16.5132712518442));
#8960=CARTESIAN_POINT('',(0.822592072616804,-2.,16.5132712518442));
#8961=CARTESIAN_POINT('',(-0.653797257879687,-2.,9.5675146666121));
#8962=CARTESIAN_POINT('',(0.822592072616804,-4.,16.5132712518442));
#8963=CARTESIAN_POINT('',(-0.653797257879687,-4.,9.5675146666121));
#8964=CARTESIAN_POINT('',(0.822592072616806,-2.,16.5132712518442));
#8965=CARTESIAN_POINT('Origin',(-0.248714874327312,-2.,9.44225746837724));
#8966=CARTESIAN_POINT('',(-0.248714874327312,-2.,9.44225746837724));
#8967=CARTESIAN_POINT('',(-0.248714874327312,-4.,9.44225746837724));
#8968=CARTESIAN_POINT('Origin',(5.11429163215176E-16,-2.,42.));
#8969=CARTESIAN_POINT('',(-2.25911010841498,-4.,16.600267294358));
#8970=CARTESIAN_POINT('Origin',(5.11429163215176E-16,-4.,42.));
#8971=CARTESIAN_POINT('',(-2.25911010841498,-2.,16.600267294358));
#8972=CARTESIAN_POINT('',(-2.25911010841497,-2.,16.600267294358));
#8973=CARTESIAN_POINT('Origin',(5.11429163215176E-16,-2.,42.));
#8974=CARTESIAN_POINT('Origin',(-7.38260308224823,-2.,10.4121743786501));
#8975=CARTESIAN_POINT('',(-7.01241515654904,-2.,10.2054329874371));
#8976=CARTESIAN_POINT('',(-7.38260308224823,-2.,10.4121743786501));
#8977=CARTESIAN_POINT('',(-7.01241515654904,-2.,10.2054329874371));
#8978=CARTESIAN_POINT('',(-7.01241515654904,-4.,10.2054329874371));
#8979=CARTESIAN_POINT('',(-7.01241515654904,-2.,10.2054329874371));
#8980=CARTESIAN_POINT('',(-7.38260308224823,-4.,10.4121743786501));
#8981=CARTESIAN_POINT('',(-7.01241515654904,-4.,10.2054329874371));
#8982=CARTESIAN_POINT('',(-7.38260308224823,-2.,10.4121743786501));
#8983=CARTESIAN_POINT('Origin',(-4.49437240522989,-2.,16.8991909157671));
#8984=CARTESIAN_POINT('',(-4.49437240522989,-2.,16.8991909157671));
#8985=CARTESIAN_POINT('',(-7.38260308224823,-2.,10.4121743786501));
#8986=CARTESIAN_POINT('',(-4.49437240522989,-4.,16.8991909157671));
#8987=CARTESIAN_POINT('',(-7.38260308224823,-4.,10.4121743786501));
#8988=CARTESIAN_POINT('',(-4.49437240522989,-2.,16.8991909157671));
#8989=CARTESIAN_POINT('Origin',(-7.01241515654904,-2.,10.2054329874371));
#8990=CARTESIAN_POINT('',(-7.01241515654904,-2.,10.2054329874371));
#8991=CARTESIAN_POINT('',(-7.01241515654904,-4.,10.2054329874371));
#8992=CARTESIAN_POINT('Origin',(5.11429163215176E-16,-2.,42.));
#8993=CARTESIAN_POINT('',(-7.49064450548875,-4.,17.6250077970804));
#8994=CARTESIAN_POINT('Origin',(5.11429163215176E-16,-4.,42.));
#8995=CARTESIAN_POINT('',(-7.49064450548875,-2.,17.6250077970804));
#8996=CARTESIAN_POINT('',(-7.49064450548876,-2.,17.6250077970804));
#8997=CARTESIAN_POINT('Origin',(5.11429163215176E-16,-2.,42.));
#8998=CARTESIAN_POINT('Origin',(-28.41425483552,-2.,26.3499623675545));
#8999=CARTESIAN_POINT('',(-28.3201895594221,-2.,25.9365221336551));
#9000=CARTESIAN_POINT('',(-28.41425483552,-2.,26.3499623675545));
#9001=CARTESIAN_POINT('',(-28.3201895594221,-2.,25.9365221336551));
#9002=CARTESIAN_POINT('',(-28.3201895594221,-4.,25.9365221336551));
#9003=CARTESIAN_POINT('',(-28.3201895594221,-2.,25.9365221336551));
#9004=CARTESIAN_POINT('',(-28.41425483552,-4.,26.3499623675545));
#9005=CARTESIAN_POINT('',(-28.3201895594221,-4.,25.9365221336551));
#9006=CARTESIAN_POINT('',(-28.41425483552,-2.,26.3499623675545));
#9007=CARTESIAN_POINT('Origin',(-21.6608585189576,-2.,28.5442499940843));
#9008=CARTESIAN_POINT('',(-21.6608585189576,-2.,28.5442499940843));
#9009=CARTESIAN_POINT('',(-28.41425483552,-2.,26.3499623675545));
#9010=CARTESIAN_POINT('',(-21.6608585189576,-4.,28.5442499940843));
#9011=CARTESIAN_POINT('',(-28.41425483552,-4.,26.3499623675545));
#9012=CARTESIAN_POINT('',(-21.6608585189576,-2.,28.5442499940843));
#9013=CARTESIAN_POINT('Origin',(-28.3201895594221,-2.,25.9365221336551));
#9014=CARTESIAN_POINT('',(-20.3873196453819,-2.,26.6831074405731));
#9015=CARTESIAN_POINT('',(-28.3201895594221,-2.,25.9365221336551));
#9016=CARTESIAN_POINT('',(-20.3873196453819,-4.,26.6831074405731));
#9017=CARTESIAN_POINT('',(-20.3873196453819,-2.,26.6831074405731));
#9018=CARTESIAN_POINT('',(-28.3201895594221,-4.,25.9365221336551));
#9019=CARTESIAN_POINT('Origin',(5.11429163215176E-16,-2.,42.));
#9020=CARTESIAN_POINT('',(-23.1263688266279,-4.,31.2565803910126));
#9021=CARTESIAN_POINT('Origin',(5.11429163215176E-16,-4.,42.));
#9022=CARTESIAN_POINT('',(-23.1263688266279,-2.,31.2565803910126));
#9023=CARTESIAN_POINT('',(-23.1263688266279,-2.,31.2565803910126));
#9024=CARTESIAN_POINT('Origin',(5.11429163215176E-16,-2.,42.));
#9025=CARTESIAN_POINT('Origin',(5.11429163215176E-16,-2.,42.));
#9026=CARTESIAN_POINT('',(-18.3899090552018,-2.,24.3347446963989));
#9027=CARTESIAN_POINT('Origin',(5.11429163215176E-16,-2.,42.));
#9028=CARTESIAN_POINT('',(-18.3899090552018,-4.,24.3347446963989));
#9029=CARTESIAN_POINT('',(-18.3899090552018,-2.,24.3347446963989));
#9030=CARTESIAN_POINT('Origin',(5.11429163215176E-16,-4.,42.));
#9031=CARTESIAN_POINT('Origin',(-13.7887537262625,-2.,12.6373736455454));
#9032=CARTESIAN_POINT('',(-13.4696392471283,-2.,12.3581836522056));
#9033=CARTESIAN_POINT('',(-13.7887537262625,-2.,12.6373736455454));
#9034=CARTESIAN_POINT('',(-13.4696392471283,-2.,12.3581836522056));
#9035=CARTESIAN_POINT('',(-13.4696392471283,-4.,12.3581836522056));
#9036=CARTESIAN_POINT('',(-13.4696392471283,-2.,12.3581836522056));
#9037=CARTESIAN_POINT('',(-13.7887537262625,-4.,12.6373736455454));
#9038=CARTESIAN_POINT('',(-13.4696392471283,-4.,12.3581836522056));
#9039=CARTESIAN_POINT('',(-13.7887537262625,-2.,12.6373736455454));
#9040=CARTESIAN_POINT('Origin',(-9.61491124257647,-2.,18.3821363837163));
#9041=CARTESIAN_POINT('',(-9.61491124257647,-2.,18.3821363837163));
#9042=CARTESIAN_POINT('',(-13.7887537262625,-2.,12.6373736455454));
#9043=CARTESIAN_POINT('',(-9.61491124257647,-4.,18.3821363837163));
#9044=CARTESIAN_POINT('',(-13.7887537262625,-4.,12.6373736455454));
#9045=CARTESIAN_POINT('',(-9.61491124257647,-2.,18.3821363837163));
#9046=CARTESIAN_POINT('Origin',(-13.4696392471283,-2.,12.3581836522056));
#9047=CARTESIAN_POINT('',(-13.4696392471283,-2.,12.3581836522056));
#9048=CARTESIAN_POINT('',(-13.4696392471283,-4.,12.3581836522056));
#9049=CARTESIAN_POINT('Origin',(5.11429163215176E-16,-2.,42.));
#9050=CARTESIAN_POINT('',(-12.3948017935724,-4.,19.7150524232599));
#9051=CARTESIAN_POINT('Origin',(5.11429163215176E-16,-4.,42.));
#9052=CARTESIAN_POINT('',(-12.3948017935724,-2.,19.7150524232599));
#9053=CARTESIAN_POINT('',(-12.3948017935724,-2.,19.7150524232599));
#9054=CARTESIAN_POINT('Origin',(5.11429163215176E-16,-2.,42.));
#9055=CARTESIAN_POINT('Origin',(-19.5922696666578,-2.,16.1458605816439));
#9056=CARTESIAN_POINT('',(-19.3381754681079,-2.,15.8064239285885));
#9057=CARTESIAN_POINT('',(-19.5922696666578,-2.,16.1458605816439));
#9058=CARTESIAN_POINT('',(-19.3381754681079,-2.,15.8064239285885));
#9059=CARTESIAN_POINT('',(-19.3381754681079,-4.,15.8064239285885));
#9060=CARTESIAN_POINT('',(-19.3381754681079,-2.,15.8064239285885));
#9061=CARTESIAN_POINT('',(-19.5922696666578,-4.,16.1458605816439));
#9062=CARTESIAN_POINT('',(-19.3381754681079,-4.,15.8064239285885));
#9063=CARTESIAN_POINT('',(-19.5922696666578,-2.,16.1458605816439));
#9064=CARTESIAN_POINT('Origin',(-14.3152323211595,-2.,20.8972958227806));
#9065=CARTESIAN_POINT('',(-14.3152323211595,-2.,20.8972958227806));
#9066=CARTESIAN_POINT('',(-19.5922696666578,-2.,16.1458605816439));
#9067=CARTESIAN_POINT('',(-14.3152323211595,-4.,20.8972958227806));
#9068=CARTESIAN_POINT('',(-19.5922696666578,-4.,16.1458605816439));
#9069=CARTESIAN_POINT('',(-14.3152323211594,-2.,20.8972958227806));
#9070=CARTESIAN_POINT('Origin',(-19.3381754681079,-2.,15.8064239285885));
#9071=CARTESIAN_POINT('',(-19.3381754681079,-2.,15.8064239285885));
#9072=CARTESIAN_POINT('',(-19.3381754681079,-4.,15.8064239285885));
#9073=CARTESIAN_POINT('Origin',(5.11429163215176E-16,-2.,42.));
#9074=CARTESIAN_POINT('',(-16.7572467664191,-4.,22.7790561935857));
#9075=CARTESIAN_POINT('Origin',(5.11429163215176E-16,-4.,42.));
#9076=CARTESIAN_POINT('',(-16.7572467664191,-2.,22.7790561935857));
#9077=CARTESIAN_POINT('',(-16.7572467664191,-2.,22.7790561935857));
#9078=CARTESIAN_POINT('Origin',(5.11429163215176E-16,-2.,42.));
#9079=CARTESIAN_POINT('Origin',(-24.5395094084795,-2.,20.78429747225));
#9080=CARTESIAN_POINT('',(-24.3615406262698,-2.,20.3994491700153));
#9081=CARTESIAN_POINT('',(-24.5395094084795,-2.,20.78429747225));
#9082=CARTESIAN_POINT('',(-24.3615406262698,-2.,20.3994491700153));
#9083=CARTESIAN_POINT('',(-24.3615406262698,-4.,20.3994491700153));
#9084=CARTESIAN_POINT('',(-24.3615406262698,-2.,20.3994491700153));
#9085=CARTESIAN_POINT('',(-24.5395094084795,-4.,20.78429747225));
#9086=CARTESIAN_POINT('',(-24.3615406262698,-4.,20.3994491700153));
#9087=CARTESIAN_POINT('',(-24.5395094084795,-2.,20.78429747225));
#9088=CARTESIAN_POINT('Origin',(-18.3899090552018,-2.,24.3347446963989));
#9089=CARTESIAN_POINT('',(-24.5395094084795,-2.,20.78429747225));
#9090=CARTESIAN_POINT('',(-24.5395094084795,-4.,20.78429747225));
#9091=CARTESIAN_POINT('Origin',(-24.3615406262698,-2.,20.3994491700153));
#9092=CARTESIAN_POINT('',(-24.3615406262698,-2.,20.3994491700153));
#9093=CARTESIAN_POINT('',(-24.3615406262698,-4.,20.3994491700153));
#9094=CARTESIAN_POINT('Origin',(-32.3231572079194,-2.,39.2600978362433));
#9095=CARTESIAN_POINT('',(-32.405385595067,-2.,38.8441415939278));
#9096=CARTESIAN_POINT('',(-32.3231572079194,-2.,39.2600978362433));
#9097=CARTESIAN_POINT('',(-32.405385595067,-2.,38.8441415939278));
#9098=CARTESIAN_POINT('',(-32.405385595067,-4.,38.8441415939278));
#9099=CARTESIAN_POINT('',(-32.405385595067,-2.,38.8441415939278));
#9100=CARTESIAN_POINT('',(-32.3231572079194,-4.,39.2600978362433));
#9101=CARTESIAN_POINT('',(-32.405385595067,-4.,38.8441415939278));
#9102=CARTESIAN_POINT('',(-32.3231572079194,-2.,39.2600978362433));
#9103=CARTESIAN_POINT('Origin',(-25.2611254961061,-2.,38.517825583062));
#9104=CARTESIAN_POINT('',(-25.2611254961061,-2.,38.517825583062));
#9105=CARTESIAN_POINT('',(-32.3231572079194,-2.,39.2600978362433));
#9106=CARTESIAN_POINT('',(-25.2611254961061,-4.,38.517825583062));
#9107=CARTESIAN_POINT('',(-32.3231572079194,-4.,39.2600978362433));
#9108=CARTESIAN_POINT('',(-25.2611254961061,-2.,38.517825583062));
#9109=CARTESIAN_POINT('Origin',(-32.405385595067,-2.,38.8441415939278));
#9110=CARTESIAN_POINT('',(-24.8546847175204,-2.,36.2995923310118));
#9111=CARTESIAN_POINT('',(-32.405385595067,-2.,38.8441415939278));
#9112=CARTESIAN_POINT('',(-24.8546847175204,-4.,36.2995923310118));
#9113=CARTESIAN_POINT('',(-24.8546847175204,-2.,36.2995923310118));
#9114=CARTESIAN_POINT('',(-32.405385595067,-4.,38.8441415939278));
#9115=CARTESIAN_POINT('Origin',(5.11429163215176E-16,-2.,42.));
#9116=CARTESIAN_POINT('',(-25.4967316202476,-4.,41.5917394397366));
#9117=CARTESIAN_POINT('Origin',(5.11429163215176E-16,-4.,42.));
#9118=CARTESIAN_POINT('',(-25.4967316202476,-2.,41.5917394397366));
#9119=CARTESIAN_POINT('',(-25.4967316202476,-2.,41.5917394397366));
#9120=CARTESIAN_POINT('Origin',(5.11429163215176E-16,-2.,42.));
#9121=CARTESIAN_POINT('Origin',(5.11429163215176E-16,-2.,42.));
#9122=CARTESIAN_POINT('',(-23.9851245251038,-2.,33.3418361348804));
#9123=CARTESIAN_POINT('Origin',(5.11429163215176E-16,-2.,42.));
#9124=CARTESIAN_POINT('',(-23.9851245251038,-4.,33.3418361348804));
#9125=CARTESIAN_POINT('',(-23.9851245251038,-2.,33.3418361348804));
#9126=CARTESIAN_POINT('Origin',(5.11429163215176E-16,-4.,42.));
#9127=CARTESIAN_POINT('Origin',(-31.0471609795261,-2.,32.5996090046093));
#9128=CARTESIAN_POINT('',(-31.0411103134807,-2.,32.1756461611731));
#9129=CARTESIAN_POINT('',(-31.0471609795261,-2.,32.5996090046093));
#9130=CARTESIAN_POINT('',(-31.0411103134807,-2.,32.1756461611731));
#9131=CARTESIAN_POINT('',(-31.0411103134807,-4.,32.1756461611731));
#9132=CARTESIAN_POINT('',(-31.0411103134807,-2.,32.1756461611731));
#9133=CARTESIAN_POINT('',(-31.0471609795261,-4.,32.5996090046093));
#9134=CARTESIAN_POINT('',(-31.0411103134807,-4.,32.1756461611731));
#9135=CARTESIAN_POINT('',(-31.0471609795261,-2.,32.5996090046093));
#9136=CARTESIAN_POINT('Origin',(-23.9851245251038,-2.,33.3418361348804));
#9137=CARTESIAN_POINT('',(-31.0471609795261,-2.,32.5996090046093));
#9138=CARTESIAN_POINT('',(-31.0471609795261,-4.,32.5996090046093));
#9139=CARTESIAN_POINT('Origin',(-31.0411103134807,-2.,32.1756461611731));
#9140=CARTESIAN_POINT('',(-31.0411103134807,-2.,32.1756461611731));
#9141=CARTESIAN_POINT('',(-31.0411103134807,-4.,32.1756461611731));
#9142=CARTESIAN_POINT('Origin',(7.38260308224823,-2.,73.5878256213499));
#9143=CARTESIAN_POINT('',(7.01241515654905,-2.,73.7945670125629));
#9144=CARTESIAN_POINT('',(7.38260308224823,-2.,73.5878256213499));
#9145=CARTESIAN_POINT('',(7.01241515654905,-2.,73.7945670125629));
#9146=CARTESIAN_POINT('',(7.01241515654905,-4.,73.7945670125629));
#9147=CARTESIAN_POINT('',(7.01241515654905,-2.,73.7945670125629));
#9148=CARTESIAN_POINT('',(7.38260308224823,-4.,73.5878256213499));
#9149=CARTESIAN_POINT('',(7.01241515654905,-4.,73.7945670125629));
#9150=CARTESIAN_POINT('',(7.38260308224823,-2.,73.5878256213499));
#9151=CARTESIAN_POINT('Origin',(4.49437240522989,-2.,67.1008090842329));
#9152=CARTESIAN_POINT('',(4.49437240522989,-2.,67.1008090842329));
#9153=CARTESIAN_POINT('',(7.38260308224823,-2.,73.5878256213499));
#9154=CARTESIAN_POINT('',(4.49437240522989,-4.,67.1008090842329));
#9155=CARTESIAN_POINT('',(7.38260308224823,-4.,73.5878256213499));
#9156=CARTESIAN_POINT('',(4.49437240522989,-2.,67.1008090842329));
#9157=CARTESIAN_POINT('Origin',(7.01241515654905,-2.,73.7945670125629));
#9158=CARTESIAN_POINT('',(2.25911010841498,-2.,67.399732705642));
#9159=CARTESIAN_POINT('',(7.01241515654905,-2.,73.7945670125629));
#9160=CARTESIAN_POINT('',(2.25911010841498,-4.,67.399732705642));
#9161=CARTESIAN_POINT('',(2.25911010841497,-2.,67.399732705642));
#9162=CARTESIAN_POINT('',(7.01241515654905,-4.,73.7945670125629));
#9163=CARTESIAN_POINT('Origin',(5.11429163215176E-16,-2.,42.));
#9164=CARTESIAN_POINT('',(7.49064450548876,-4.,66.3749922029196));
#9165=CARTESIAN_POINT('Origin',(5.11429163215176E-16,-4.,42.));
#9166=CARTESIAN_POINT('',(7.49064450548876,-2.,66.3749922029196));
#9167=CARTESIAN_POINT('',(7.49064450548877,-2.,66.3749922029196));
#9168=CARTESIAN_POINT('Origin',(5.11429163215176E-16,-2.,42.));
#9169=CARTESIAN_POINT('Origin',(5.11429163215176E-16,-2.,42.));
#9170=CARTESIAN_POINT('',(-0.822592072616806,-2.,67.4867287481558));
#9171=CARTESIAN_POINT('Origin',(5.11429163215176E-16,-2.,42.));
#9172=CARTESIAN_POINT('',(-0.822592072616806,-4.,67.4867287481558));
#9173=CARTESIAN_POINT('',(-0.822592072616808,-2.,67.4867287481558));
#9174=CARTESIAN_POINT('Origin',(5.11429163215176E-16,-4.,42.));
#9175=CARTESIAN_POINT('Origin',(13.7887537262625,-2.,71.3626263544546));
#9176=CARTESIAN_POINT('',(13.4696392471283,-2.,71.6418163477944));
#9177=CARTESIAN_POINT('',(13.7887537262625,-2.,71.3626263544546));
#9178=CARTESIAN_POINT('',(13.4696392471283,-2.,71.6418163477944));
#9179=CARTESIAN_POINT('',(13.4696392471283,-4.,71.6418163477944));
#9180=CARTESIAN_POINT('',(13.4696392471283,-2.,71.6418163477944));
#9181=CARTESIAN_POINT('',(13.7887537262625,-4.,71.3626263544546));
#9182=CARTESIAN_POINT('',(13.4696392471283,-4.,71.6418163477944));
#9183=CARTESIAN_POINT('',(13.7887537262625,-2.,71.3626263544546));
#9184=CARTESIAN_POINT('Origin',(9.61491124257648,-2.,65.6178636162837));
#9185=CARTESIAN_POINT('',(13.7887537262625,-2.,71.3626263544546));
#9186=CARTESIAN_POINT('',(13.7887537262625,-4.,71.3626263544546));
#9187=CARTESIAN_POINT('Origin',(13.4696392471283,-2.,71.6418163477944));
#9188=CARTESIAN_POINT('',(13.4696392471283,-2.,71.6418163477944));
#9189=CARTESIAN_POINT('',(13.4696392471283,-4.,71.6418163477944));
#9190=CARTESIAN_POINT('Origin',(-18.5344034816569,-2.,68.622724190698));
#9191=CARTESIAN_POINT('',(-18.9357463479386,-2.,68.4859579417222));
#9192=CARTESIAN_POINT('',(-18.5344034816569,-2.,68.622724190698));
#9193=CARTESIAN_POINT('',(-18.9357463479386,-2.,68.4859579417222));
#9194=CARTESIAN_POINT('',(-18.9357463479386,-4.,68.4859579417222));
#9195=CARTESIAN_POINT('',(-18.9357463479386,-2.,68.4859579417222));
#9196=CARTESIAN_POINT('',(-18.5344034816569,-4.,68.622724190698));
#9197=CARTESIAN_POINT('',(-18.9357463479386,-4.,68.4859579417222));
#9198=CARTESIAN_POINT('',(-18.5344034816569,-2.,68.622724190698));
#9199=CARTESIAN_POINT('Origin',(-15.6462142535297,-2.,62.1356891993457));
#9200=CARTESIAN_POINT('',(-15.6462142535297,-2.,62.1356891993457));
#9201=CARTESIAN_POINT('',(-18.5344034816569,-2.,68.622724190698));
#9202=CARTESIAN_POINT('',(-15.6462142535297,-4.,62.1356891993457));
#9203=CARTESIAN_POINT('',(-18.5344034816569,-4.,68.622724190698));
#9204=CARTESIAN_POINT('',(-15.6462142535297,-2.,62.1356891993457));
#9205=CARTESIAN_POINT('Origin',(-18.9357463479386,-2.,68.4859579417222));
#9206=CARTESIAN_POINT('',(-17.3640402120316,-2.,60.6745845339314));
#9207=CARTESIAN_POINT('',(-18.9357463479386,-2.,68.4859579417222));
#9208=CARTESIAN_POINT('',(-17.3640402120316,-4.,60.6745845339314));
#9209=CARTESIAN_POINT('',(-17.3640402120316,-2.,60.6745845339314));
#9210=CARTESIAN_POINT('',(-18.9357463479386,-4.,68.4859579417222));
#9211=CARTESIAN_POINT('Origin',(5.11429163215176E-16,-2.,42.));
#9212=CARTESIAN_POINT('',(-13.1019298266752,-4.,63.8766870164767));
#9213=CARTESIAN_POINT('Origin',(5.11429163215176E-16,-4.,42.));
#9214=CARTESIAN_POINT('',(-13.1019298266752,-2.,63.8766870164767));
#9215=CARTESIAN_POINT('',(-13.1019298266752,-2.,63.8766870164767));
#9216=CARTESIAN_POINT('Origin',(5.11429163215176E-16,-2.,42.));
#9217=CARTESIAN_POINT('Origin',(5.11429163215176E-16,-2.,42.));
#9218=CARTESIAN_POINT('',(-19.490752119874,-2.,58.4426452191133));
#9219=CARTESIAN_POINT('Origin',(5.11429163215176E-16,-2.,42.));
#9220=CARTESIAN_POINT('',(-19.490752119874,-4.,58.4426452191133));
#9221=CARTESIAN_POINT('',(-19.490752119874,-2.,58.4426452191133));
#9222=CARTESIAN_POINT('Origin',(5.11429163215176E-16,-4.,42.));
#9223=CARTESIAN_POINT('Origin',(-12.5942066959522,-2.,71.8944729582989));
#9224=CARTESIAN_POINT('',(-13.0152145597486,-2.,71.8441392539282));
#9225=CARTESIAN_POINT('',(-12.5942066959522,-2.,71.8944729582989));
#9226=CARTESIAN_POINT('',(-13.0152145597486,-2.,71.8441392539282));
#9227=CARTESIAN_POINT('',(-13.0152145597486,-4.,71.8441392539282));
#9228=CARTESIAN_POINT('',(-13.0152145597486,-2.,71.8441392539282));
#9229=CARTESIAN_POINT('',(-12.5942066959522,-4.,71.8944729582989));
#9230=CARTESIAN_POINT('',(-13.0152145597486,-4.,71.8441392539282));
#9231=CARTESIAN_POINT('',(-12.5942066959522,-2.,71.8944729582989));
#9232=CARTESIAN_POINT('Origin',(-11.1178617454403,-2.,64.9487069398099));
#9233=CARTESIAN_POINT('',(-11.1178617454403,-2.,64.9487069398099));
#9234=CARTESIAN_POINT('',(-12.5942066959522,-2.,71.8944729582989));
#9235=CARTESIAN_POINT('',(-11.1178617454403,-4.,64.9487069398099));
#9236=CARTESIAN_POINT('',(-12.5942066959522,-4.,71.8944729582989));
#9237=CARTESIAN_POINT('',(-11.1178617454403,-2.,64.9487069398099));
#9238=CARTESIAN_POINT('Origin',(-13.0152145597486,-2.,71.8441392539282));
#9239=CARTESIAN_POINT('',(-13.0152145597486,-2.,71.8441392539282));
#9240=CARTESIAN_POINT('',(-13.0152145597486,-4.,71.8441392539282));
#9241=CARTESIAN_POINT('Origin',(5.11429163215176E-16,-2.,42.));
#9242=CARTESIAN_POINT('',(-8.26720223785845,-4.,66.1226733004107));
#9243=CARTESIAN_POINT('Origin',(5.11429163215176E-16,-4.,42.));
#9244=CARTESIAN_POINT('',(-8.26720223785845,-2.,66.1226733004107));
#9245=CARTESIAN_POINT('',(-8.26720223785845,-2.,66.1226733004107));
#9246=CARTESIAN_POINT('Origin',(5.11429163215176E-16,-2.,42.));
#9247=CARTESIAN_POINT('Origin',(-6.1035826439255,-2.,73.8596898080255));
#9248=CARTESIAN_POINT('',(-6.5258554413689,-2.,73.8979884726687));
#9249=CARTESIAN_POINT('',(-6.1035826439255,-2.,73.8596898080255));
#9250=CARTESIAN_POINT('',(-6.5258554413689,-2.,73.8979884726687));
#9251=CARTESIAN_POINT('',(-6.5258554413689,-4.,73.8979884726687));
#9252=CARTESIAN_POINT('',(-6.5258554413689,-2.,73.8979884726687));
#9253=CARTESIAN_POINT('',(-6.1035826439255,-4.,73.8596898080255));
#9254=CARTESIAN_POINT('',(-6.5258554413689,-4.,73.8979884726687));
#9255=CARTESIAN_POINT('',(-6.1035826439255,-2.,73.8596898080255));
#9256=CARTESIAN_POINT('Origin',(-6.10360532965543,-2.,66.7587560668908));
#9257=CARTESIAN_POINT('',(-6.10360532965543,-2.,66.7587560668908));
#9258=CARTESIAN_POINT('',(-6.1035826439255,-2.,73.8596898080255));
#9259=CARTESIAN_POINT('',(-6.10360532965543,-4.,66.7587560668908));
#9260=CARTESIAN_POINT('',(-6.1035826439255,-4.,73.8596898080255));
#9261=CARTESIAN_POINT('',(-6.10360532965543,-2.,66.7587560668908));
#9262=CARTESIAN_POINT('Origin',(-6.5258554413689,-2.,73.8979884726687));
#9263=CARTESIAN_POINT('',(-6.5258554413689,-2.,73.8979884726687));
#9264=CARTESIAN_POINT('',(-6.5258554413689,-4.,73.8979884726687));
#9265=CARTESIAN_POINT('Origin',(5.11429163215176E-16,-2.,42.));
#9266=CARTESIAN_POINT('',(-3.07115824080958,-4.,67.3143830076877));
#9267=CARTESIAN_POINT('Origin',(5.11429163215176E-16,-4.,42.));
#9268=CARTESIAN_POINT('',(-3.07115824080958,-2.,67.3143830076877));
#9269=CARTESIAN_POINT('',(-3.07115824080957,-2.,67.3143830076877));
#9270=CARTESIAN_POINT('Origin',(5.11429163215176E-16,-2.,42.));
#9271=CARTESIAN_POINT('Origin',(-23.6645578972779,-2.,64.1874346259592));
#9272=CARTESIAN_POINT('',(-24.0286951569316,-2.,63.9702131737359));
#9273=CARTESIAN_POINT('',(-23.6645578972779,-2.,64.1874346259592));
#9274=CARTESIAN_POINT('',(-24.0286951569316,-2.,63.9702131737359));
#9275=CARTESIAN_POINT('',(-24.0286951569316,-4.,63.9702131737359));
#9276=CARTESIAN_POINT('',(-24.0286951569316,-2.,63.9702131737359));
#9277=CARTESIAN_POINT('',(-23.6645578972779,-4.,64.1874346259592));
#9278=CARTESIAN_POINT('',(-24.0286951569316,-4.,63.9702131737359));
#9279=CARTESIAN_POINT('',(-23.6645578972779,-2.,64.1874346259592));
#9280=CARTESIAN_POINT('Origin',(-19.490752119874,-2.,58.4426452191133));
#9281=CARTESIAN_POINT('',(-23.6645578972779,-2.,64.1874346259592));
#9282=CARTESIAN_POINT('',(-23.6645578972779,-4.,64.1874346259592));
#9283=CARTESIAN_POINT('Origin',(-24.0286951569316,-2.,63.9702131737359));
#9284=CARTESIAN_POINT('',(-20.8672587182129,-2.,56.6563130966546));
#9285=CARTESIAN_POINT('',(-24.0286951569316,-2.,63.9702131737359));
#9286=CARTESIAN_POINT('',(-20.8672587182129,-4.,56.6563130966546));
#9287=CARTESIAN_POINT('',(-20.8672587182129,-2.,56.6563130966546));
#9288=CARTESIAN_POINT('',(-24.0286951569316,-4.,63.9702131737359));
#9289=CARTESIAN_POINT('Origin',(5.11429163215176E-16,-2.,42.));
#9290=CARTESIAN_POINT('',(-22.4834505915744,-2.,54.03097874224));
#9291=CARTESIAN_POINT('Origin',(5.11429163215176E-16,-2.,42.));
#9292=CARTESIAN_POINT('',(-22.4834505915744,-4.,54.03097874224));
#9293=CARTESIAN_POINT('',(-22.4834505915744,-2.,54.03097874224));
#9294=CARTESIAN_POINT('Origin',(5.11429163215176E-16,-4.,42.));
#9295=CARTESIAN_POINT('Origin',(-30.643092052405,-2.,52.6439872802755));
#9296=CARTESIAN_POINT('',(-30.8873960676387,-2.,52.297437642684));
#9297=CARTESIAN_POINT('',(-30.643092052405,-2.,52.6439872802755));
#9298=CARTESIAN_POINT('',(-30.8873960676387,-2.,52.297437642684));
#9299=CARTESIAN_POINT('',(-30.8873960676387,-4.,52.297437642684));
#9300=CARTESIAN_POINT('',(-30.8873960676387,-2.,52.297437642684));
#9301=CARTESIAN_POINT('',(-30.643092052405,-4.,52.6439872802755));
#9302=CARTESIAN_POINT('',(-30.8873960676387,-4.,52.297437642684));
#9303=CARTESIAN_POINT('',(-30.643092052405,-2.,52.6439872802755));
#9304=CARTESIAN_POINT('Origin',(-24.4935143848573,-2.,49.0935007632897));
#9305=CARTESIAN_POINT('',(-24.4935143848573,-2.,49.0935007632897));
#9306=CARTESIAN_POINT('',(-30.643092052405,-2.,52.6439872802755));
#9307=CARTESIAN_POINT('',(-24.4935143848573,-4.,49.0935007632897));
#9308=CARTESIAN_POINT('',(-30.643092052405,-4.,52.6439872802755));
#9309=CARTESIAN_POINT('',(-24.4935143848572,-2.,49.0935007632897));
#9310=CARTESIAN_POINT('Origin',(-30.8873960676387,-2.,52.297437642684));
#9311=CARTESIAN_POINT('',(-25.0244490042775,-2.,46.9017294939964));
#9312=CARTESIAN_POINT('',(-30.8873960676387,-2.,52.297437642684));
#9313=CARTESIAN_POINT('',(-25.0244490042775,-4.,46.9017294939964));
#9314=CARTESIAN_POINT('',(-25.0244490042775,-2.,46.9017294939964));
#9315=CARTESIAN_POINT('',(-30.8873960676387,-4.,52.297437642684));
#9316=CARTESIAN_POINT('Origin',(5.11429163215176E-16,-2.,42.));
#9317=CARTESIAN_POINT('',(-23.4584778861915,-4.,51.9974904482608));
#9318=CARTESIAN_POINT('Origin',(5.11429163215176E-16,-4.,42.));
#9319=CARTESIAN_POINT('',(-23.4584778861915,-2.,51.9974904482608));
#9320=CARTESIAN_POINT('',(-23.4584778861915,-2.,51.9974904482608));
#9321=CARTESIAN_POINT('Origin',(5.11429163215176E-16,-2.,42.));
#9322=CARTESIAN_POINT('Origin',(5.11429163215176E-16,-2.,42.));
#9323=CARTESIAN_POINT('',(-25.4330940665997,-2.,43.8460027625905));
#9324=CARTESIAN_POINT('Origin',(5.11429163215176E-16,-2.,42.));
#9325=CARTESIAN_POINT('',(-25.4330940665997,-4.,43.8460027625905));
#9326=CARTESIAN_POINT('',(-25.4330940665997,-2.,43.8460027625905));
#9327=CARTESIAN_POINT('Origin',(5.11429163215176E-16,-4.,42.));
#9328=CARTESIAN_POINT('Origin',(-27.7604575776403,-2.,58.7824477009424));
#9329=CARTESIAN_POINT('',(-28.0714746850947,-2.,58.4942646652779));
#9330=CARTESIAN_POINT('',(-27.7604575776403,-2.,58.7824477009424));
#9331=CARTESIAN_POINT('',(-28.0714746850947,-2.,58.4942646652779));
#9332=CARTESIAN_POINT('',(-28.0714746850947,-4.,58.4942646652779));
#9333=CARTESIAN_POINT('',(-28.0714746850947,-2.,58.4942646652779));
#9334=CARTESIAN_POINT('',(-27.7604575776403,-4.,58.7824477009424));
#9335=CARTESIAN_POINT('',(-28.0714746850947,-4.,58.4942646652779));
#9336=CARTESIAN_POINT('',(-27.7604575776403,-2.,58.7824477009424));
#9337=CARTESIAN_POINT('Origin',(-22.4834505915744,-2.,54.03097874224));
#9338=CARTESIAN_POINT('',(-27.7604575776403,-2.,58.7824477009424));
#9339=CARTESIAN_POINT('',(-27.7604575776403,-4.,58.7824477009424));
#9340=CARTESIAN_POINT('Origin',(-28.0714746850947,-2.,58.4942646652779));
#9341=CARTESIAN_POINT('',(-28.0714746850947,-2.,58.4942646652779));
#9342=CARTESIAN_POINT('',(-28.0714746850947,-4.,58.4942646652779));
#9343=CARTESIAN_POINT('Origin',(-32.1864763626099,-2.,46.0403335399428));
#9344=CARTESIAN_POINT('',(-32.3533900278565,-2.,45.6505631825167));
#9345=CARTESIAN_POINT('',(-32.1864763626099,-2.,46.0403335399428));
#9346=CARTESIAN_POINT('',(-32.3533900278565,-2.,45.6505631825167));
#9347=CARTESIAN_POINT('',(-32.3533900278565,-4.,45.6505631825167));
#9348=CARTESIAN_POINT('',(-32.3533900278565,-2.,45.6505631825167));
#9349=CARTESIAN_POINT('',(-32.1864763626099,-4.,46.0403335399428));
#9350=CARTESIAN_POINT('',(-32.3533900278565,-4.,45.6505631825167));
#9351=CARTESIAN_POINT('',(-32.1864763626099,-2.,46.0403335399428));
#9352=CARTESIAN_POINT('Origin',(-25.4330940665997,-2.,43.8460027625905));
#9353=CARTESIAN_POINT('',(-32.1864763626099,-2.,46.0403335399428));
#9354=CARTESIAN_POINT('',(-32.1864763626099,-4.,46.0403335399428));
#9355=CARTESIAN_POINT('Origin',(-32.3533900278565,-2.,45.6505631825167));
#9356=CARTESIAN_POINT('',(-32.3533900278565,-2.,45.6505631825167));
#9357=CARTESIAN_POINT('',(-32.3533900278565,-4.,45.6505631825167));
#9358=CARTESIAN_POINT('Origin',(0.653797257879684,-2.,74.4324853333879));
#9359=CARTESIAN_POINT('',(0.248714874327309,-2.,74.5577425316228));
#9360=CARTESIAN_POINT('',(0.653797257879684,-2.,74.4324853333879));
#9361=CARTESIAN_POINT('',(0.248714874327309,-2.,74.5577425316228));
#9362=CARTESIAN_POINT('',(0.248714874327309,-4.,74.5577425316228));
#9363=CARTESIAN_POINT('',(0.248714874327309,-2.,74.5577425316228));
#9364=CARTESIAN_POINT('',(0.653797257879684,-4.,74.4324853333879));
#9365=CARTESIAN_POINT('',(0.248714874327309,-4.,74.5577425316228));
#9366=CARTESIAN_POINT('',(0.653797257879684,-2.,74.4324853333879));
#9367=CARTESIAN_POINT('Origin',(-0.822592072616806,-2.,67.4867287481558));
#9368=CARTESIAN_POINT('',(0.653797257879684,-2.,74.4324853333879));
#9369=CARTESIAN_POINT('',(0.653797257879684,-4.,74.4324853333879));
#9370=CARTESIAN_POINT('Origin',(0.248714874327309,-2.,74.5577425316228));
#9371=CARTESIAN_POINT('',(0.248714874327309,-2.,74.5577425316228));
#9372=CARTESIAN_POINT('',(0.248714874327309,-4.,74.5577425316228));
#9373=CARTESIAN_POINT('Origin',(21.9692735008546,-2.,43.1623346526058));
#9374=CARTESIAN_POINT('',(6.705461117593,-2.,44.0091767469411));
#9375=CARTESIAN_POINT('',(21.9692735008546,-2.,43.1623346526058));
#9376=CARTESIAN_POINT('',(6.705461117593,-2.,44.0091767469411));
#9377=CARTESIAN_POINT('',(6.705461117593,-4.,44.0091767469411));
#9378=CARTESIAN_POINT('',(6.70546111759299,-2.,44.0091767469411));
#9379=CARTESIAN_POINT('',(21.9692735008546,-4.,43.1623346526058));
#9380=CARTESIAN_POINT('',(6.705461117593,-4.,44.0091767469411));
#9381=CARTESIAN_POINT('',(21.9692735008546,-2.,43.1623346526058));
#9382=CARTESIAN_POINT('Origin',(6.705461117593,-2.,39.9908232530589));
#9383=CARTESIAN_POINT('',(6.705461117593,-2.,39.9908232530589));
#9384=CARTESIAN_POINT('',(21.9692735008546,-2.,40.8376653473942));
#9385=CARTESIAN_POINT('',(6.705461117593,-2.,39.9908232530589));
#9386=CARTESIAN_POINT('',(21.9692735008546,-4.,40.8376653473942));
#9387=CARTESIAN_POINT('',(21.9692735008546,-2.,40.8376653473942));
#9388=CARTESIAN_POINT('',(6.705461117593,-4.,39.9908232530589));
#9389=CARTESIAN_POINT('',(6.705461117593,-4.,39.9908232530589));
#9390=CARTESIAN_POINT('',(6.705461117593,-2.,39.9908232530589));
#9391=CARTESIAN_POINT('Origin',(5.11429163215176E-16,-2.,42.));
#9392=CARTESIAN_POINT('',(11.9912480872829,-4.,60.4447816281255));
#9393=CARTESIAN_POINT('Origin',(5.11429163215176E-16,-4.,42.));
#9394=CARTESIAN_POINT('',(11.9912480872829,-2.,60.4447816281255));
#9395=CARTESIAN_POINT('',(11.9912480872829,-2.,60.4447816281255));
#9396=CARTESIAN_POINT('Origin',(5.11429163215176E-16,-2.,42.));
#9397=CARTESIAN_POINT('Origin',(5.11429163215176E-16,-2.,42.));
#9398=CARTESIAN_POINT('',(11.9912480872829,-2.,23.5552183718745));
#9399=CARTESIAN_POINT('Origin',(5.11429163215176E-16,-2.,42.));
#9400=CARTESIAN_POINT('',(11.9912480872829,-4.,23.5552183718745));
#9401=CARTESIAN_POINT('',(11.9912480872829,-2.,23.5552183718745));
#9402=CARTESIAN_POINT('Origin',(5.11429163215176E-16,-4.,42.));
#9403=CARTESIAN_POINT('Origin',(5.11429163215176E-16,-2.,42.));
#9404=CARTESIAN_POINT('',(5.09272866234044,-4.,37.1974887015462));
#9405=CARTESIAN_POINT('Origin',(5.11429163215176E-16,-4.,42.));
#9406=CARTESIAN_POINT('',(5.09272866234044,-2.,37.1974887015462));
#9407=CARTESIAN_POINT('',(5.09272866234044,-2.,37.1974887015462));
#9408=CARTESIAN_POINT('Origin',(5.11429163215176E-16,-2.,42.));
#9409=CARTESIAN_POINT('Origin',(5.11429163215176E-16,-2.,42.));
#9410=CARTESIAN_POINT('',(5.09272866234043,-2.,46.8025112984538));
#9411=CARTESIAN_POINT('Origin',(5.11429163215176E-16,-2.,42.));
#9412=CARTESIAN_POINT('',(5.09272866234043,-4.,46.8025112984538));
#9413=CARTESIAN_POINT('',(5.09272866234043,-2.,46.8025112984538));
#9414=CARTESIAN_POINT('Origin',(5.11429163215176E-16,-4.,42.));
#9415=CARTESIAN_POINT('Origin',(11.9912480872829,-2.,23.5552183718745));
#9416=CARTESIAN_POINT('',(5.09272866234044,-2.,37.1974887015462));
#9417=CARTESIAN_POINT('',(5.09272866234044,-4.,37.1974887015462));
#9418=CARTESIAN_POINT('Origin',(1.61273245525256,-2.,35.1883119546051));
#9419=CARTESIAN_POINT('',(1.61273245525256,-2.,35.1883119546051));
#9420=CARTESIAN_POINT('',(9.97802541357168,-2.,22.3928837192687));
#9421=CARTESIAN_POINT('',(1.61273245525256,-2.,35.1883119546051));
#9422=CARTESIAN_POINT('',(9.97802541357168,-4.,22.3928837192687));
#9423=CARTESIAN_POINT('',(9.97802541357168,-2.,22.3928837192687));
#9424=CARTESIAN_POINT('',(1.61273245525256,-4.,35.1883119546051));
#9425=CARTESIAN_POINT('',(1.61273245525256,-4.,35.1883119546051));
#9426=CARTESIAN_POINT('',(1.61273245525256,-2.,35.1883119546051));
#9427=CARTESIAN_POINT('Origin',(5.11429163215176E-16,-2.,42.));
#9428=CARTESIAN_POINT('',(-9.97802541357168,-2.,22.3928837192687));
#9429=CARTESIAN_POINT('Origin',(5.11429163215176E-16,-2.,42.));
#9430=CARTESIAN_POINT('',(-9.97802541357168,-4.,22.3928837192687));
#9431=CARTESIAN_POINT('',(-9.97802541357167,-2.,22.3928837192687));
#9432=CARTESIAN_POINT('Origin',(5.11429163215176E-16,-4.,42.));
#9433=CARTESIAN_POINT('Origin',(5.11429163215176E-16,-2.,42.));
#9434=CARTESIAN_POINT('',(-1.61273245525256,-4.,35.1883119546051));
#9435=CARTESIAN_POINT('Origin',(5.11429163215176E-16,-4.,42.));
#9436=CARTESIAN_POINT('',(-1.61273245525256,-2.,35.1883119546051));
#9437=CARTESIAN_POINT('',(-1.61273245525255,-2.,35.1883119546051));
#9438=CARTESIAN_POINT('Origin',(5.11429163215176E-16,-2.,42.));
#9439=CARTESIAN_POINT('Origin',(-9.97802541357168,-2.,22.3928837192687));
#9440=CARTESIAN_POINT('',(-1.61273245525256,-2.,35.1883119546051));
#9441=CARTESIAN_POINT('',(-1.61273245525256,-4.,35.1883119546051));
#9442=CARTESIAN_POINT('Origin',(-5.09272866234044,-2.,37.1974887015462));
#9443=CARTESIAN_POINT('',(-5.09272866234044,-2.,37.1974887015462));
#9444=CARTESIAN_POINT('',(-11.9912480872829,-2.,23.5552183718745));
#9445=CARTESIAN_POINT('',(-5.09272866234044,-2.,37.1974887015462));
#9446=CARTESIAN_POINT('',(-11.9912480872829,-4.,23.5552183718745));
#9447=CARTESIAN_POINT('',(-11.9912480872829,-2.,23.5552183718745));
#9448=CARTESIAN_POINT('',(-5.09272866234044,-4.,37.1974887015462));
#9449=CARTESIAN_POINT('',(-5.09272866234044,-4.,37.1974887015462));
#9450=CARTESIAN_POINT('',(-5.09272866234043,-2.,37.1974887015462));
#9451=CARTESIAN_POINT('Origin',(5.11429163215176E-16,-2.,42.));
#9452=CARTESIAN_POINT('',(-21.9692735008546,-2.,40.8376653473942));
#9453=CARTESIAN_POINT('Origin',(5.11429163215176E-16,-2.,42.));
#9454=CARTESIAN_POINT('',(-21.9692735008546,-4.,40.8376653473942));
#9455=CARTESIAN_POINT('',(-21.9692735008546,-2.,40.8376653473942));
#9456=CARTESIAN_POINT('Origin',(5.11429163215176E-16,-4.,42.));
#9457=CARTESIAN_POINT('Origin',(5.11429163215176E-16,-2.,42.));
#9458=CARTESIAN_POINT('',(-6.705461117593,-4.,39.9908232530589));
#9459=CARTESIAN_POINT('Origin',(5.11429163215176E-16,-4.,42.));
#9460=CARTESIAN_POINT('',(-6.705461117593,-2.,39.9908232530589));
#9461=CARTESIAN_POINT('',(-6.70546111759299,-2.,39.9908232530589));
#9462=CARTESIAN_POINT('Origin',(5.11429163215176E-16,-2.,42.));
#9463=CARTESIAN_POINT('Origin',(-21.9692735008546,-2.,40.8376653473942));
#9464=CARTESIAN_POINT('',(-6.705461117593,-2.,39.9908232530589));
#9465=CARTESIAN_POINT('',(-6.705461117593,-4.,39.9908232530589));
#9466=CARTESIAN_POINT('Origin',(-6.705461117593,-2.,44.0091767469411));
#9467=CARTESIAN_POINT('',(-6.705461117593,-2.,44.0091767469411));
#9468=CARTESIAN_POINT('',(-21.9692735008546,-2.,43.1623346526058));
#9469=CARTESIAN_POINT('',(-6.705461117593,-2.,44.0091767469411));
#9470=CARTESIAN_POINT('',(-21.9692735008546,-4.,43.1623346526058));
#9471=CARTESIAN_POINT('',(-21.9692735008546,-2.,43.1623346526058));
#9472=CARTESIAN_POINT('',(-6.705461117593,-4.,44.0091767469411));
#9473=CARTESIAN_POINT('',(-6.705461117593,-4.,44.0091767469411));
#9474=CARTESIAN_POINT('',(-6.70546111759299,-2.,44.0091767469411));
#9475=CARTESIAN_POINT('Origin',(5.11429163215176E-16,-2.,42.));
#9476=CARTESIAN_POINT('',(-11.9912480872829,-2.,60.4447816281255));
#9477=CARTESIAN_POINT('Origin',(5.11429163215176E-16,-2.,42.));
#9478=CARTESIAN_POINT('',(-11.9912480872829,-4.,60.4447816281255));
#9479=CARTESIAN_POINT('',(-11.9912480872829,-2.,60.4447816281255));
#9480=CARTESIAN_POINT('Origin',(5.11429163215176E-16,-4.,42.));
#9481=CARTESIAN_POINT('Origin',(5.11429163215176E-16,-2.,42.));
#9482=CARTESIAN_POINT('',(-5.09272866234044,-4.,46.8025112984538));
#9483=CARTESIAN_POINT('Origin',(5.11429163215176E-16,-4.,42.));
#9484=CARTESIAN_POINT('',(-5.09272866234044,-2.,46.8025112984538));
#9485=CARTESIAN_POINT('',(-5.09272866234044,-2.,46.8025112984538));
#9486=CARTESIAN_POINT('Origin',(5.11429163215176E-16,-2.,42.));
#9487=CARTESIAN_POINT('Origin',(-11.9912480872829,-2.,60.4447816281255));
#9488=CARTESIAN_POINT('',(-5.09272866234044,-2.,46.8025112984538));
#9489=CARTESIAN_POINT('',(-5.09272866234044,-4.,46.8025112984538));
#9490=CARTESIAN_POINT('Origin',(-1.61273245525257,-2.,48.8116880453949));
#9491=CARTESIAN_POINT('',(-1.61273245525257,-2.,48.8116880453949));
#9492=CARTESIAN_POINT('',(-9.97802541357169,-2.,61.6071162807313));
#9493=CARTESIAN_POINT('',(-1.61273245525257,-2.,48.8116880453949));
#9494=CARTESIAN_POINT('',(-9.97802541357169,-4.,61.6071162807313));
#9495=CARTESIAN_POINT('',(-9.97802541357169,-2.,61.6071162807313));
#9496=CARTESIAN_POINT('',(-1.61273245525257,-4.,48.8116880453949));
#9497=CARTESIAN_POINT('',(-1.61273245525257,-4.,48.8116880453949));
#9498=CARTESIAN_POINT('',(-1.61273245525256,-2.,48.8116880453949));
#9499=CARTESIAN_POINT('Origin',(5.11429163215176E-16,-2.,42.));
#9500=CARTESIAN_POINT('',(9.97802541357166,-2.,61.6071162807313));
#9501=CARTESIAN_POINT('Origin',(5.11429163215176E-16,-2.,42.));
#9502=CARTESIAN_POINT('',(9.97802541357166,-4.,61.6071162807313));
#9503=CARTESIAN_POINT('',(9.97802541357166,-2.,61.6071162807313));
#9504=CARTESIAN_POINT('Origin',(5.11429163215176E-16,-4.,42.));
#9505=CARTESIAN_POINT('Origin',(5.11429163215176E-16,-2.,42.));
#9506=CARTESIAN_POINT('',(1.61273245525255,-4.,48.8116880453949));
#9507=CARTESIAN_POINT('Origin',(5.11429163215176E-16,-4.,42.));
#9508=CARTESIAN_POINT('',(1.61273245525255,-2.,48.8116880453949));
#9509=CARTESIAN_POINT('',(1.61273245525255,-2.,48.8116880453949));
#9510=CARTESIAN_POINT('Origin',(5.11429163215176E-16,-2.,42.));
#9511=CARTESIAN_POINT('Origin',(9.97802541357166,-2.,61.6071162807313));
#9512=CARTESIAN_POINT('',(1.61273245525255,-2.,48.8116880453949));
#9513=CARTESIAN_POINT('',(1.61273245525255,-4.,48.8116880453949));
#9514=CARTESIAN_POINT('Origin',(5.09272866234043,-2.,46.8025112984538));
#9515=CARTESIAN_POINT('',(5.09272866234043,-2.,46.8025112984538));
#9516=CARTESIAN_POINT('',(5.09272866234043,-4.,46.8025112984538));
#9517=CARTESIAN_POINT('Origin',(5.11429163215176E-16,-2.,42.));
#9518=CARTESIAN_POINT('',(-6.00000000000001,-2.,42.));
#9519=CARTESIAN_POINT('Origin',(5.11429163215176E-16,-2.,42.));
#9520=CARTESIAN_POINT('',(-6.00000000000001,-4.,42.));
#9521=CARTESIAN_POINT('',(-6.00000000000001,-2.,42.));
#9522=CARTESIAN_POINT('Origin',(5.11429163215176E-16,-4.,42.));
#9523=CARTESIAN_POINT('Origin',(0.,-4.,42.));
#9524=CARTESIAN_POINT('Origin',(0.,-2.,42.));
#9878=UNCERTAINTY_MEASURE_WITH_UNIT(LENGTH_MEASURE(0.01),#9892,
'DISTANCE_ACCURACY_VALUE',
'Maximum model space distance between geometric entities at asserted c
onnectivities');
#9881=UNCERTAINTY_MEASURE_WITH_UNIT(LENGTH_MEASURE(0.01),#9892,
'DISTANCE_ACCURACY_VALUE',
'Maximum model space distance between geometric entities at asserted c
onnectivities');
#9888=(
GEOMETRIC_REPRESENTATION_CONTEXT(3)
GLOBAL_UNCERTAINTY_ASSIGNED_CONTEXT((#9878))
GLOBAL_UNIT_ASSIGNED_CONTEXT((#9892,#9894,#9895))
REPRESENTATION_CONTEXT('','3D')
);
#9891=(
GEOMETRIC_REPRESENTATION_CONTEXT(3)
GLOBAL_UNCERTAINTY_ASSIGNED_CONTEXT((#9881))
GLOBAL_UNIT_ASSIGNED_CONTEXT((#9892,#9894,#9895))
REPRESENTATION_CONTEXT('','3D')
);
#9892=(
LENGTH_UNIT()
NAMED_UNIT(*)
SI_UNIT(.MILLI.,.METRE.)
);
#9894=(
NAMED_UNIT(*)
PLANE_ANGLE_UNIT()
SI_UNIT($,.RADIAN.)
);
#9895=(
NAMED_UNIT(*)
SI_UNIT($,.STERADIAN.)
SOLID_ANGLE_UNIT()
);
#9902=SHAPE_DEFINITION_REPRESENTATION(#9911,#9928);
#9911=PRODUCT_DEFINITION_SHAPE('',$,#9938);
#9928=SHAPE_REPRESENTATION('',(#5948),#9888);
#9931=PRODUCT_DEFINITION_CONTEXT('part definition',#9960,'design');
#9938=PRODUCT_DEFINITION('Wheel','Wheel',#9947,#9931);
#9947=PRODUCT_DEFINITION_FORMATION('',$,#9968);
#9960=APPLICATION_CONTEXT(
'Core Data for Automotive Mechanical Design Process');
#9961=PRODUCT_CONTEXT('part definition',#9960,'mechanical');
#9968=PRODUCT('Wheel','Wheel',$,(#9961));
#9974=PRESENTATION_STYLE_ASSIGNMENT((#9979));
#9979=SURFACE_STYLE_USAGE(.BOTH.,#9984);
#9984=SURFACE_SIDE_STYLE('',(#9989));
#9989=SURFACE_STYLE_FILL_AREA(#9994);
#9994=FILL_AREA_STYLE('Opaque(255,242,183)',(#9999));
#9999=FILL_AREA_STYLE_COLOUR('Opaque(255,242,183)',#10004);
#10004=COLOUR_RGB('Opaque(255,242,183)', 0.08235294, 0.09019608, 0.10196078);
ENDSEC;
END-ISO-10303-21;
